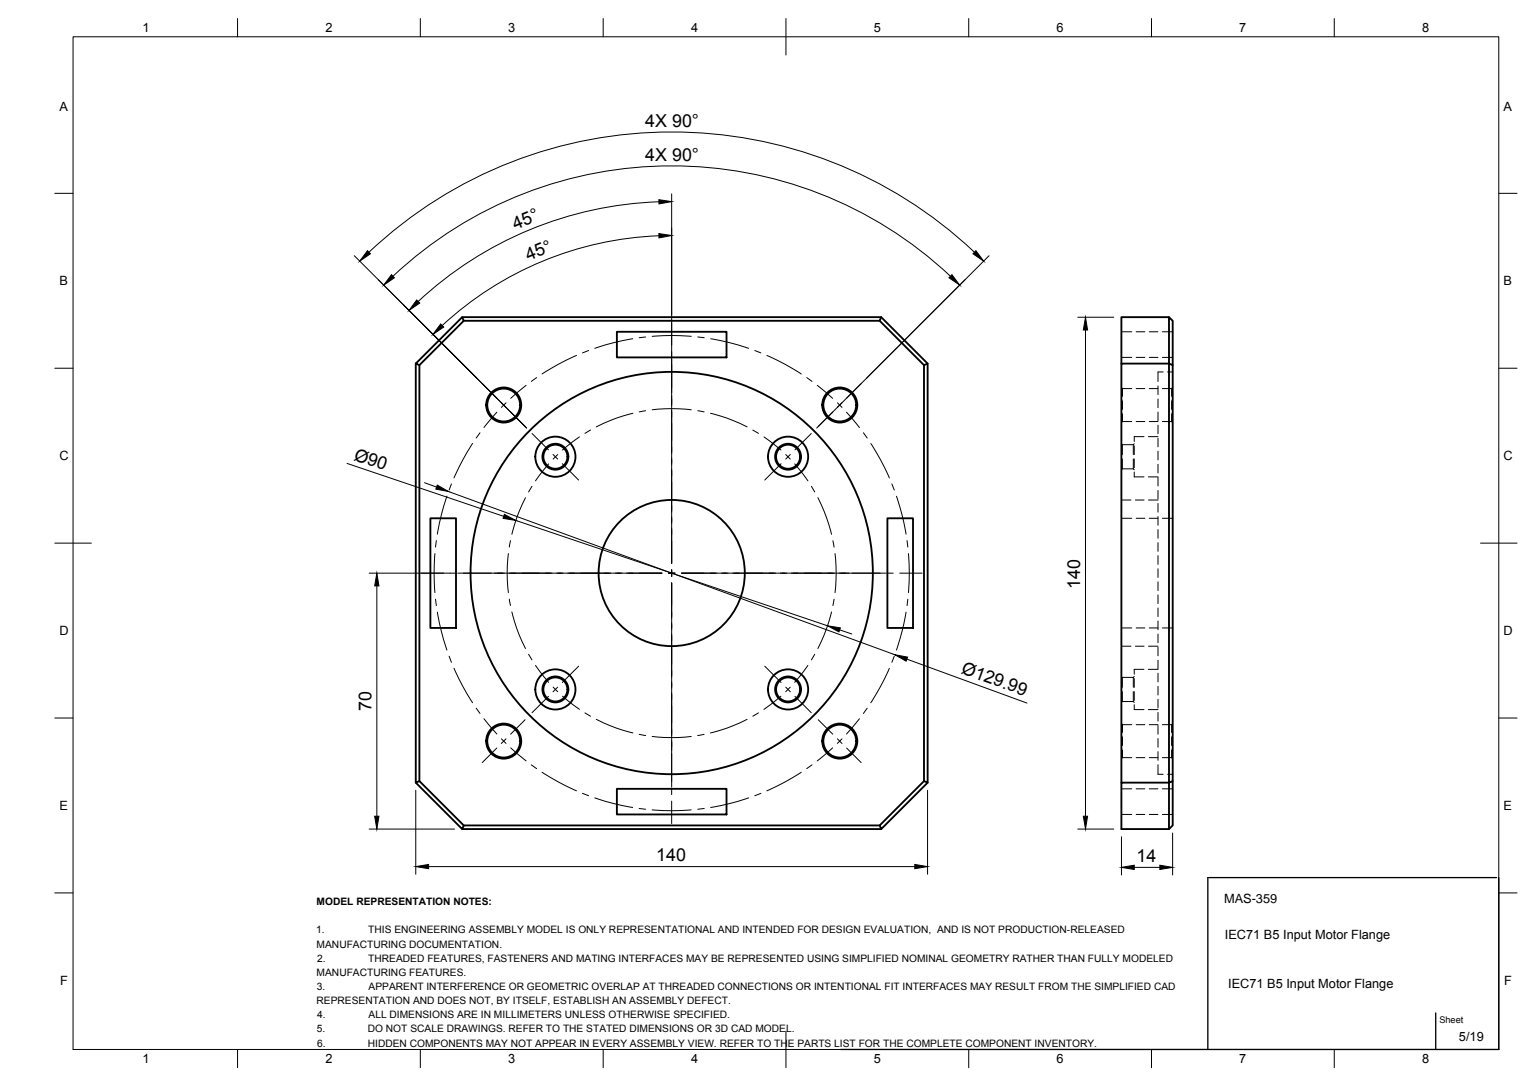
ISO-10303-21;
HEADER;
/* Generated by software containing ST-Developer
 * from STEP Tools, Inc. (www.steptools.com) 
 */

FILE_DESCRIPTION(
/* description */ (''),
/* implementation_level */ '2;1');

FILE_NAME(
/* name */ 'IEC71 B5 Input Motor Flange.step',
/* time_stamp */ '2026-10-15T14:25:16-07:00',
/* author */ (''),
/* organization */ (''),
/* preprocessor_version */ 'ST-DEVELOPER v20.2',
/* originating_system */ 'Autodesk Translation Framework v15.15.0.0',
/* authorisation */ '');

FILE_SCHEMA (('AUTOMOTIVE_DESIGN { 1 0 10303 214 3 1 1 }'));
ENDSEC;

DATA;
#10=MECHANICAL_DESIGN_GEOMETRIC_PRESENTATION_REPRESENTATION('',(#325),#86429);
#289=SHAPE_REPRESENTATION_RELATIONSHIP('SRR','None',#86504,#307);
#307=ADVANCED_BREP_SHAPE_REPRESENTATION('',(#343),#86413);
#325=STYLED_ITEM('',(#86603),#343);
#343=MANIFOLD_SOLID_BREP('Body1',#15615);
#1211=CONICAL_SURFACE('',#16324,0.3425,0.321750554396649);
#1212=CONICAL_SURFACE('',#16329,0.3425,0.785398163397466);
#1213=CONICAL_SURFACE('',#16335,0.3425,0.321750554396644);
#1214=CONICAL_SURFACE('',#16340,0.3425,0.785398163397457);
#1215=CONICAL_SURFACE('',#16346,0.3425,0.321750554396649);
#1216=CONICAL_SURFACE('',#16351,0.3425,0.785398163397466);
#1217=CONICAL_SURFACE('',#16357,0.3425,0.321750554396644);
#1218=CONICAL_SURFACE('',#16362,0.3425,0.785398163397457);
#1219=CONICAL_SURFACE('',#16368,0.49,0.785398163397448);
#1220=CONICAL_SURFACE('',#16373,0.49,0.785398163397443);
#1221=CONICAL_SURFACE('',#16374,0.49,0.785398163397448);
#1222=CONICAL_SURFACE('',#16379,0.49,0.785398163397443);
#1223=CONICAL_SURFACE('',#16380,0.49,0.785398163397448);
#1224=CONICAL_SURFACE('',#16385,0.49,0.785398163397443);
#1225=CONICAL_SURFACE('',#16386,0.49,0.785398163397448);
#1226=CONICAL_SURFACE('',#16391,0.49,0.785398163397443);
#1418=CYLINDRICAL_SURFACE('',#16327,0.33);
#1419=CYLINDRICAL_SURFACE('',#16333,0.55);
#1420=CYLINDRICAL_SURFACE('',#16338,0.33);
#1421=CYLINDRICAL_SURFACE('',#16344,0.55);
#1422=CYLINDRICAL_SURFACE('',#16349,0.33);
#1423=CYLINDRICAL_SURFACE('',#16355,0.55);
#1424=CYLINDRICAL_SURFACE('',#16360,0.33);
#1425=CYLINDRICAL_SURFACE('',#16366,0.55);
#1426=CYLINDRICAL_SURFACE('',#16371,0.45);
#1427=CYLINDRICAL_SURFACE('',#16377,0.45);
#1428=CYLINDRICAL_SURFACE('',#16383,0.45);
#1429=CYLINDRICAL_SURFACE('',#16389,0.45);
#1430=CYLINDRICAL_SURFACE('',#16408,2.);
#1431=CYLINDRICAL_SURFACE('',#16411,5.501);
#1668=FACE_BOUND('',#3613,.T.);
#1669=FACE_BOUND('',#3614,.T.);
#1670=FACE_BOUND('',#3615,.T.);
#1671=FACE_BOUND('',#3616,.T.);
#1672=FACE_BOUND('',#3617,.T.);
#1673=FACE_BOUND('',#3618,.T.);
#1674=FACE_BOUND('',#3619,.T.);
#1675=FACE_BOUND('',#3620,.T.);
#1676=FACE_BOUND('',#3621,.T.);
#1677=FACE_BOUND('',#3626,.T.);
#1678=FACE_BOUND('',#3632,.T.);
#1679=FACE_BOUND('',#3638,.T.);
#1680=FACE_BOUND('',#3644,.T.);
#1681=FACE_BOUND('',#3677,.T.);
#1682=FACE_BOUND('',#3678,.T.);
#1683=FACE_BOUND('',#3679,.T.);
#1684=FACE_BOUND('',#3680,.T.);
#1685=FACE_BOUND('',#3681,.T.);
#1686=FACE_BOUND('',#3687,.T.);
#1687=FACE_BOUND('',#3688,.T.);
#1688=FACE_BOUND('',#3689,.T.);
#1689=FACE_BOUND('',#3690,.T.);
#1690=FACE_BOUND('',#3691,.T.);
#1691=FACE_BOUND('',#3692,.T.);
#1692=FACE_BOUND('',#3693,.T.);
#1693=FACE_BOUND('',#3694,.T.);
#1694=FACE_BOUND('',#3695,.T.);
#1695=FACE_BOUND('',#3696,.T.);
#1696=FACE_BOUND('',#3697,.T.);
#1697=FACE_BOUND('',#3698,.T.);
#1698=FACE_BOUND('',#3699,.T.);
#1945=CIRCLE('',#16319,0.480000000000001);
#1946=CIRCLE('',#16320,5.501);
#1947=CIRCLE('',#16321,0.480000000000001);
#1948=CIRCLE('',#16322,0.480000000000001);
#1949=CIRCLE('',#16323,0.480000000000001);
#1950=CIRCLE('',#16325,0.33);
#1951=CIRCLE('',#16326,0.338333333333333);
#1952=CIRCLE('',#16328,0.33);
#1953=CIRCLE('',#16330,0.355);
#1954=CIRCLE('',#16332,0.55);
#1955=CIRCLE('',#16334,0.55);
#1956=CIRCLE('',#16336,0.33);
#1957=CIRCLE('',#16337,0.338333333333333);
#1958=CIRCLE('',#16339,0.33);
#1959=CIRCLE('',#16341,0.355);
#1960=CIRCLE('',#16343,0.55);
#1961=CIRCLE('',#16345,0.55);
#1962=CIRCLE('',#16347,0.33);
#1963=CIRCLE('',#16348,0.338333333333333);
#1964=CIRCLE('',#16350,0.33);
#1965=CIRCLE('',#16352,0.355);
#1966=CIRCLE('',#16354,0.55);
#1967=CIRCLE('',#16356,0.55);
#1968=CIRCLE('',#16358,0.33);
#1969=CIRCLE('',#16359,0.338333333333333);
#1970=CIRCLE('',#16361,0.33);
#1971=CIRCLE('',#16363,0.355);
#1972=CIRCLE('',#16365,0.55);
#1973=CIRCLE('',#16367,0.55);
#1974=CIRCLE('',#16369,0.45);
#1975=CIRCLE('',#16370,0.48);
#1976=CIRCLE('',#16372,0.45);
#1977=CIRCLE('',#16375,0.45);
#1978=CIRCLE('',#16376,0.48);
#1979=CIRCLE('',#16378,0.45);
#1980=CIRCLE('',#16381,0.45);
#1981=CIRCLE('',#16382,0.48);
#1982=CIRCLE('',#16384,0.45);
#1983=CIRCLE('',#16387,0.45);
#1984=CIRCLE('',#16388,0.48);
#1985=CIRCLE('',#16390,0.45);
#1986=CIRCLE('',#16409,2.);
#1987=CIRCLE('',#16410,2.);
#1988=CIRCLE('',#16412,5.501);
#2662=FACE_OUTER_BOUND('',#3600,.T.);
#2663=FACE_OUTER_BOUND('',#3601,.T.);
#2664=FACE_OUTER_BOUND('',#3602,.T.);
#2665=FACE_OUTER_BOUND('',#3603,.T.);
#2666=FACE_OUTER_BOUND('',#3604,.T.);
#2667=FACE_OUTER_BOUND('',#3605,.T.);
#2668=FACE_OUTER_BOUND('',#3606,.T.);
#2669=FACE_OUTER_BOUND('',#3607,.T.);
#2670=FACE_OUTER_BOUND('',#3608,.T.);
#2671=FACE_OUTER_BOUND('',#3609,.T.);
#2672=FACE_OUTER_BOUND('',#3610,.T.);
#2673=FACE_OUTER_BOUND('',#3611,.T.);
#2674=FACE_OUTER_BOUND('',#3612,.T.);
#2675=FACE_OUTER_BOUND('',#3622,.T.);
#2676=FACE_OUTER_BOUND('',#3623,.T.);
#2677=FACE_OUTER_BOUND('',#3624,.T.);
#2678=FACE_OUTER_BOUND('',#3625,.T.);
#2679=FACE_OUTER_BOUND('',#3627,.T.);
#2680=FACE_OUTER_BOUND('',#3628,.T.);
#2681=FACE_OUTER_BOUND('',#3629,.T.);
#2682=FACE_OUTER_BOUND('',#3630,.T.);
#2683=FACE_OUTER_BOUND('',#3631,.T.);
#2684=FACE_OUTER_BOUND('',#3633,.T.);
#2685=FACE_OUTER_BOUND('',#3634,.T.);
#2686=FACE_OUTER_BOUND('',#3635,.T.);
#2687=FACE_OUTER_BOUND('',#3636,.T.);
#2688=FACE_OUTER_BOUND('',#3637,.T.);
#2689=FACE_OUTER_BOUND('',#3639,.T.);
#2690=FACE_OUTER_BOUND('',#3640,.T.);
#2691=FACE_OUTER_BOUND('',#3641,.T.);
#2692=FACE_OUTER_BOUND('',#3642,.T.);
#2693=FACE_OUTER_BOUND('',#3643,.T.);
#2694=FACE_OUTER_BOUND('',#3645,.T.);
#2695=FACE_OUTER_BOUND('',#3646,.T.);
#2696=FACE_OUTER_BOUND('',#3647,.T.);
#2697=FACE_OUTER_BOUND('',#3648,.T.);
#2698=FACE_OUTER_BOUND('',#3649,.T.);
#2699=FACE_OUTER_BOUND('',#3650,.T.);
#2700=FACE_OUTER_BOUND('',#3651,.T.);
#2701=FACE_OUTER_BOUND('',#3652,.T.);
#2702=FACE_OUTER_BOUND('',#3653,.T.);
#2703=FACE_OUTER_BOUND('',#3654,.T.);
#2704=FACE_OUTER_BOUND('',#3655,.T.);
#2705=FACE_OUTER_BOUND('',#3656,.T.);
#2706=FACE_OUTER_BOUND('',#3657,.T.);
#2707=FACE_OUTER_BOUND('',#3658,.T.);
#2708=FACE_OUTER_BOUND('',#3659,.T.);
#2709=FACE_OUTER_BOUND('',#3660,.T.);
#2710=FACE_OUTER_BOUND('',#3661,.T.);
#2711=FACE_OUTER_BOUND('',#3662,.T.);
#2712=FACE_OUTER_BOUND('',#3663,.T.);
#2713=FACE_OUTER_BOUND('',#3664,.T.);
#2714=FACE_OUTER_BOUND('',#3665,.T.);
#2715=FACE_OUTER_BOUND('',#3666,.T.);
#2716=FACE_OUTER_BOUND('',#3667,.T.);
#2717=FACE_OUTER_BOUND('',#3668,.T.);
#2718=FACE_OUTER_BOUND('',#3669,.T.);
#2719=FACE_OUTER_BOUND('',#3670,.T.);
#2720=FACE_OUTER_BOUND('',#3671,.T.);
#2721=FACE_OUTER_BOUND('',#3672,.T.);
#2722=FACE_OUTER_BOUND('',#3673,.T.);
#2723=FACE_OUTER_BOUND('',#3674,.T.);
#2724=FACE_OUTER_BOUND('',#3675,.T.);
#2725=FACE_OUTER_BOUND('',#3676,.T.);
#2726=FACE_OUTER_BOUND('',#3682,.T.);
#2727=FACE_OUTER_BOUND('',#3683,.T.);
#2728=FACE_OUTER_BOUND('',#3684,.T.);
#2729=FACE_OUTER_BOUND('',#3685,.T.);
#2730=FACE_OUTER_BOUND('',#3686,.T.);
#3600=EDGE_LOOP('',(#11207,#11208,#11209,#11210));
#3601=EDGE_LOOP('',(#11211,#11212,#11213,#11214));
#3602=EDGE_LOOP('',(#11215,#11216,#11217,#11218));
#3603=EDGE_LOOP('',(#11219,#11220,#11221,#11222));
#3604=EDGE_LOOP('',(#11223,#11224,#11225,#11226));
#3605=EDGE_LOOP('',(#11227,#11228,#11229,#11230));
#3606=EDGE_LOOP('',(#11231,#11232,#11233,#11234));
#3607=EDGE_LOOP('',(#11235,#11236,#11237,#11238));
#3608=EDGE_LOOP('',(#11239,#11240,#11241,#11242));
#3609=EDGE_LOOP('',(#11243,#11244,#11245,#11246));
#3610=EDGE_LOOP('',(#11247,#11248,#11249,#11250));
#3611=EDGE_LOOP('',(#11251,#11252,#11253,#11254));
#3612=EDGE_LOOP('',(#11255,#11256,#11257,#11258,#11259,#11260,#11261,#11262));
#3613=EDGE_LOOP('',(#11263));
#3614=EDGE_LOOP('',(#11264,#11265,#11266,#11267));
#3615=EDGE_LOOP('',(#11268,#11269,#11270,#11271));
#3616=EDGE_LOOP('',(#11272,#11273,#11274,#11275));
#3617=EDGE_LOOP('',(#11276,#11277,#11278,#11279));
#3618=EDGE_LOOP('',(#11280));
#3619=EDGE_LOOP('',(#11281));
#3620=EDGE_LOOP('',(#11282));
#3621=EDGE_LOOP('',(#11283));
#3622=EDGE_LOOP('',(#11284,#11285,#11286,#11287));
#3623=EDGE_LOOP('',(#11288,#11289,#11290,#11291));
#3624=EDGE_LOOP('',(#11292,#11293,#11294,#11295));
#3625=EDGE_LOOP('',(#11296));
#3626=EDGE_LOOP('',(#11297));
#3627=EDGE_LOOP('',(#11298,#11299,#11300,#11301));
#3628=EDGE_LOOP('',(#11302,#11303,#11304,#11305));
#3629=EDGE_LOOP('',(#11306,#11307,#11308,#11309));
#3630=EDGE_LOOP('',(#11310,#11311,#11312,#11313));
#3631=EDGE_LOOP('',(#11314));
#3632=EDGE_LOOP('',(#11315));
#3633=EDGE_LOOP('',(#11316,#11317,#11318,#11319));
#3634=EDGE_LOOP('',(#11320,#11321,#11322,#11323));
#3635=EDGE_LOOP('',(#11324,#11325,#11326,#11327));
#3636=EDGE_LOOP('',(#11328,#11329,#11330,#11331));
#3637=EDGE_LOOP('',(#11332));
#3638=EDGE_LOOP('',(#11333));
#3639=EDGE_LOOP('',(#11334,#11335,#11336,#11337));
#3640=EDGE_LOOP('',(#11338,#11339,#11340,#11341));
#3641=EDGE_LOOP('',(#11342,#11343,#11344,#11345));
#3642=EDGE_LOOP('',(#11346,#11347,#11348,#11349));
#3643=EDGE_LOOP('',(#11350));
#3644=EDGE_LOOP('',(#11351));
#3645=EDGE_LOOP('',(#11352,#11353,#11354,#11355));
#3646=EDGE_LOOP('',(#11356,#11357,#11358,#11359));
#3647=EDGE_LOOP('',(#11360,#11361,#11362,#11363));
#3648=EDGE_LOOP('',(#11364,#11365,#11366,#11367));
#3649=EDGE_LOOP('',(#11368,#11369,#11370,#11371));
#3650=EDGE_LOOP('',(#11372,#11373,#11374,#11375));
#3651=EDGE_LOOP('',(#11376,#11377,#11378,#11379));
#3652=EDGE_LOOP('',(#11380,#11381,#11382,#11383));
#3653=EDGE_LOOP('',(#11384,#11385,#11386,#11387));
#3654=EDGE_LOOP('',(#11388,#11389,#11390,#11391));
#3655=EDGE_LOOP('',(#11392,#11393,#11394,#11395));
#3656=EDGE_LOOP('',(#11396,#11397,#11398,#11399));
#3657=EDGE_LOOP('',(#11400,#11401,#11402,#11403));
#3658=EDGE_LOOP('',(#11404,#11405,#11406,#11407));
#3659=EDGE_LOOP('',(#11408,#11409,#11410,#11411));
#3660=EDGE_LOOP('',(#11412,#11413,#11414,#11415));
#3661=EDGE_LOOP('',(#11416,#11417,#11418,#11419));
#3662=EDGE_LOOP('',(#11420,#11421,#11422,#11423));
#3663=EDGE_LOOP('',(#11424,#11425,#11426,#11427));
#3664=EDGE_LOOP('',(#11428,#11429,#11430,#11431));
#3665=EDGE_LOOP('',(#11432,#11433,#11434,#11435));
#3666=EDGE_LOOP('',(#11436,#11437,#11438,#11439));
#3667=EDGE_LOOP('',(#11440,#11441,#11442,#11443));
#3668=EDGE_LOOP('',(#11444,#11445,#11446,#11447));
#3669=EDGE_LOOP('',(#11448,#11449,#11450,#11451));
#3670=EDGE_LOOP('',(#11452,#11453,#11454,#11455));
#3671=EDGE_LOOP('',(#11456,#11457,#11458,#11459));
#3672=EDGE_LOOP('',(#11460,#11461,#11462,#11463));
#3673=EDGE_LOOP('',(#11464,#11465,#11466,#11467));
#3674=EDGE_LOOP('',(#11468,#11469,#11470,#11471));
#3675=EDGE_LOOP('',(#11472,#11473,#11474,#11475));
#3676=EDGE_LOOP('',(#11476));
#3677=EDGE_LOOP('',(#11477));
#3678=EDGE_LOOP('',(#11478));
#3679=EDGE_LOOP('',(#11479));
#3680=EDGE_LOOP('',(#11480));
#3681=EDGE_LOOP('',(#11481));
#3682=EDGE_LOOP('',(#11482,#11483,#11484,#11485));
#3683=EDGE_LOOP('',(#11486,#11487,#11488,#11489));
#3684=EDGE_LOOP('',(#11490,#11491,#11492,#11493));
#3685=EDGE_LOOP('',(#11494,#11495,#11496,#11497));
#3686=EDGE_LOOP('',(#11498,#11499,#11500,#11501,#11502,#11503,#11504,#11505));
#3687=EDGE_LOOP('',(#11506));
#3688=EDGE_LOOP('',(#11507));
#3689=EDGE_LOOP('',(#11508));
#3690=EDGE_LOOP('',(#11509));
#3691=EDGE_LOOP('',(#11510));
#3692=EDGE_LOOP('',(#11511));
#3693=EDGE_LOOP('',(#11512,#11513,#11514,#11515));
#3694=EDGE_LOOP('',(#11516,#11517,#11518,#11519));
#3695=EDGE_LOOP('',(#11520,#11521,#11522,#11523));
#3696=EDGE_LOOP('',(#11524,#11525,#11526,#11527));
#3697=EDGE_LOOP('',(#11528));
#3698=EDGE_LOOP('',(#11529));
#3699=EDGE_LOOP('',(#11530));
#4732=LINE('',#22793,#5592);
#4733=LINE('',#22795,#5593);
#4734=LINE('',#22797,#5594);
#4735=LINE('',#22798,#5595);
#4736=LINE('',#22801,#5596);
#4737=LINE('',#22803,#5597);
#4738=LINE('',#22804,#5598);
#4739=LINE('',#22807,#5599);
#4740=LINE('',#22809,#5600);
#4741=LINE('',#22810,#5601);
#4742=LINE('',#22813,#5602);
#4743=LINE('',#22815,#5603);
#4744=LINE('',#22816,#5604);
#4745=LINE('',#22819,#5605);
#4746=LINE('',#22821,#5606);
#4747=LINE('',#22822,#5607);
#4748=LINE('',#22825,#5608);
#4749=LINE('',#22827,#5609);
#4750=LINE('',#22828,#5610);
#4751=LINE('',#22831,#5611);
#4752=LINE('',#22833,#5612);
#4753=LINE('',#22834,#5613);
#4754=LINE('',#22836,#5614);
#4755=LINE('',#22837,#5615);
#4756=LINE('',#22840,#5616);
#4757=LINE('',#22842,#5617);
#4758=LINE('',#22843,#5618);
#4759=LINE('',#22846,#5619);
#4760=LINE('',#22847,#5620);
#4761=LINE('',#22850,#5621);
#4762=LINE('',#22851,#5622);
#4763=LINE('',#22854,#5623);
#4764=LINE('',#22855,#5624);
#4765=LINE('',#22861,#5625);
#4766=LINE('',#22863,#5626);
#4767=LINE('',#22865,#5627);
#4768=LINE('',#22866,#5628);
#4769=LINE('',#22869,#5629);
#4770=LINE('',#22871,#5630);
#4771=LINE('',#22873,#5631);
#4772=LINE('',#22874,#5632);
#4773=LINE('',#22877,#5633);
#4774=LINE('',#22879,#5634);
#4775=LINE('',#22881,#5635);
#4776=LINE('',#22882,#5636);
#4777=LINE('',#22885,#5637);
#4778=LINE('',#22887,#5638);
#4779=LINE('',#22889,#5639);
#4780=LINE('',#22890,#5640);
#4781=LINE('',#22903,#5641);
#4782=LINE('',#22907,#5642);
#4783=LINE('',#22911,#5643);
#4784=LINE('',#22918,#5644);
#4785=LINE('',#22924,#5645);
#4786=LINE('',#22928,#5646);
#4787=LINE('',#22932,#5647);
#4788=LINE('',#22939,#5648);
#4789=LINE('',#22945,#5649);
#4790=LINE('',#22949,#5650);
#4791=LINE('',#22953,#5651);
#4792=LINE('',#22960,#5652);
#4793=LINE('',#22966,#5653);
#4794=LINE('',#22970,#5654);
#4795=LINE('',#22974,#5655);
#4796=LINE('',#22981,#5656);
#4797=LINE('',#22987,#5657);
#4798=LINE('',#22991,#5658);
#4799=LINE('',#22994,#5659);
#4800=LINE('',#22999,#5660);
#4801=LINE('',#23003,#5661);
#4802=LINE('',#23006,#5662);
#4803=LINE('',#23011,#5663);
#4804=LINE('',#23015,#5664);
#4805=LINE('',#23018,#5665);
#4806=LINE('',#23023,#5666);
#4807=LINE('',#23027,#5667);
#4808=LINE('',#23030,#5668);
#4809=LINE('',#23034,#5669);
#4810=LINE('',#23035,#5670);
#4811=LINE('',#23036,#5671);
#4812=LINE('',#23039,#5672);
#4813=LINE('',#23040,#5673);
#4814=LINE('',#23043,#5674);
#4815=LINE('',#23044,#5675);
#4816=LINE('',#23046,#5676);
#4817=LINE('',#23050,#5677);
#4818=LINE('',#23051,#5678);
#4819=LINE('',#23052,#5679);
#4820=LINE('',#23055,#5680);
#4821=LINE('',#23056,#5681);
#4822=LINE('',#23059,#5682);
#4823=LINE('',#23060,#5683);
#4824=LINE('',#23062,#5684);
#4825=LINE('',#23066,#5685);
#4826=LINE('',#23067,#5686);
#4827=LINE('',#23068,#5687);
#4828=LINE('',#23071,#5688);
#4829=LINE('',#23072,#5689);
#4830=LINE('',#23075,#5690);
#4831=LINE('',#23076,#5691);
#4832=LINE('',#23078,#5692);
#4833=LINE('',#23082,#5693);
#4834=LINE('',#23083,#5694);
#4835=LINE('',#23084,#5695);
#4836=LINE('',#23087,#5696);
#4837=LINE('',#23088,#5697);
#4838=LINE('',#23091,#5698);
#4839=LINE('',#23092,#5699);
#4840=LINE('',#23094,#5700);
#4841=LINE('',#23099,#5701);
#4842=LINE('',#23103,#5702);
#4843=LINE('',#23108,#5703);
#4844=LINE('',#23109,#5704);
#4845=LINE('',#23112,#5705);
#4846=LINE('',#23113,#5706);
#4847=LINE('',#23116,#5707);
#4848=LINE('',#23117,#5708);
#4849=LINE('',#23119,#5709);
#5592=VECTOR('',#18691,1.);
#5593=VECTOR('',#18692,1.);
#5594=VECTOR('',#18693,1.);
#5595=VECTOR('',#18694,0.999999999999999);
#5596=VECTOR('',#18697,1.);
#5597=VECTOR('',#18698,1.);
#5598=VECTOR('',#18699,1.);
#5599=VECTOR('',#18702,1.);
#5600=VECTOR('',#18703,1.);
#5601=VECTOR('',#18704,1.);
#5602=VECTOR('',#18707,1.);
#5603=VECTOR('',#18708,0.999999999999999);
#5604=VECTOR('',#18709,1.);
#5605=VECTOR('',#18712,1.);
#5606=VECTOR('',#18713,0.999999999999999);
#5607=VECTOR('',#18714,1.);
#5608=VECTOR('',#18717,1.);
#5609=VECTOR('',#18718,1.);
#5610=VECTOR('',#18719,1.);
#5611=VECTOR('',#18722,1.);
#5612=VECTOR('',#18723,1.);
#5613=VECTOR('',#18724,1.);
#5614=VECTOR('',#18727,1.);
#5615=VECTOR('',#18728,1.);
#5616=VECTOR('',#18731,1.);
#5617=VECTOR('',#18732,1.);
#5618=VECTOR('',#18733,1.);
#5619=VECTOR('',#18736,1.);
#5620=VECTOR('',#18737,1.);
#5621=VECTOR('',#18740,1.);
#5622=VECTOR('',#18741,1.);
#5623=VECTOR('',#18744,1.);
#5624=VECTOR('',#18745,1.);
#5625=VECTOR('',#18750,1.);
#5626=VECTOR('',#18751,1.);
#5627=VECTOR('',#18752,1.);
#5628=VECTOR('',#18753,1.);
#5629=VECTOR('',#18754,1.);
#5630=VECTOR('',#18755,1.);
#5631=VECTOR('',#18756,1.);
#5632=VECTOR('',#18757,1.);
#5633=VECTOR('',#18758,1.);
#5634=VECTOR('',#18759,1.);
#5635=VECTOR('',#18760,1.);
#5636=VECTOR('',#18761,1.);
#5637=VECTOR('',#18762,1.);
#5638=VECTOR('',#18763,1.);
#5639=VECTOR('',#18764,1.);
#5640=VECTOR('',#18765,1.);
#5641=VECTOR('',#18778,0.3425);
#5642=VECTOR('',#18783,0.33);
#5643=VECTOR('',#18788,0.3425);
#5644=VECTOR('',#18797,0.55);
#5645=VECTOR('',#18804,0.3425);
#5646=VECTOR('',#18809,0.33);
#5647=VECTOR('',#18814,0.3425);
#5648=VECTOR('',#18823,0.55);
#5649=VECTOR('',#18830,0.3425);
#5650=VECTOR('',#18835,0.33);
#5651=VECTOR('',#18840,0.3425);
#5652=VECTOR('',#18849,0.55);
#5653=VECTOR('',#18856,0.3425);
#5654=VECTOR('',#18861,0.33);
#5655=VECTOR('',#18866,0.3425);
#5656=VECTOR('',#18875,0.55);
#5657=VECTOR('',#18882,0.49);
#5658=VECTOR('',#18887,0.45);
#5659=VECTOR('',#18892,0.49);
#5660=VECTOR('',#18897,0.49);
#5661=VECTOR('',#18902,0.45);
#5662=VECTOR('',#18907,0.49);
#5663=VECTOR('',#18912,0.49);
#5664=VECTOR('',#18917,0.45);
#5665=VECTOR('',#18922,0.49);
#5666=VECTOR('',#18927,0.49);
#5667=VECTOR('',#18932,0.45);
#5668=VECTOR('',#18937,0.49);
#5669=VECTOR('',#18940,1.);
#5670=VECTOR('',#18941,1.);
#5671=VECTOR('',#18942,1.);
#5672=VECTOR('',#18945,1.);
#5673=VECTOR('',#18946,1.);
#5674=VECTOR('',#18949,1.);
#5675=VECTOR('',#18950,1.);
#5676=VECTOR('',#18953,1.);
#5677=VECTOR('',#18956,1.);
#5678=VECTOR('',#18957,1.);
#5679=VECTOR('',#18958,1.);
#5680=VECTOR('',#18961,1.);
#5681=VECTOR('',#18962,1.);
#5682=VECTOR('',#18965,1.);
#5683=VECTOR('',#18966,1.);
#5684=VECTOR('',#18969,1.);
#5685=VECTOR('',#18972,1.);
#5686=VECTOR('',#18973,1.);
#5687=VECTOR('',#18974,1.);
#5688=VECTOR('',#18977,1.);
#5689=VECTOR('',#18978,1.);
#5690=VECTOR('',#18981,1.);
#5691=VECTOR('',#18982,1.);
#5692=VECTOR('',#18985,1.);
#5693=VECTOR('',#18988,1.);
#5694=VECTOR('',#18989,1.);
#5695=VECTOR('',#18990,1.);
#5696=VECTOR('',#18993,1.);
#5697=VECTOR('',#18994,1.);
#5698=VECTOR('',#18997,1.);
#5699=VECTOR('',#18998,1.);
#5700=VECTOR('',#19001,1.);
#5701=VECTOR('',#19006,2.);
#5702=VECTOR('',#19011,5.501);
#5703=VECTOR('',#19018,1.);
#5704=VECTOR('',#19019,1.);
#5705=VECTOR('',#19022,1.);
#5706=VECTOR('',#19023,1.);
#5707=VECTOR('',#19026,1.);
#5708=VECTOR('',#19027,1.);
#5709=VECTOR('',#19030,1.);
#6442=VERTEX_POINT('',#22791);
#6443=VERTEX_POINT('',#22792);
#6444=VERTEX_POINT('',#22794);
#6445=VERTEX_POINT('',#22796);
#6446=VERTEX_POINT('',#22800);
#6447=VERTEX_POINT('',#22802);
#6448=VERTEX_POINT('',#22806);
#6449=VERTEX_POINT('',#22808);
#6450=VERTEX_POINT('',#22812);
#6451=VERTEX_POINT('',#22814);
#6452=VERTEX_POINT('',#22818);
#6453=VERTEX_POINT('',#22820);
#6454=VERTEX_POINT('',#22824);
#6455=VERTEX_POINT('',#22826);
#6456=VERTEX_POINT('',#22830);
#6457=VERTEX_POINT('',#22832);
#6458=VERTEX_POINT('',#22839);
#6459=VERTEX_POINT('',#22841);
#6460=VERTEX_POINT('',#22845);
#6461=VERTEX_POINT('',#22849);
#6462=VERTEX_POINT('',#22853);
#6463=VERTEX_POINT('',#22857);
#6464=VERTEX_POINT('',#22859);
#6465=VERTEX_POINT('',#22860);
#6466=VERTEX_POINT('',#22862);
#6467=VERTEX_POINT('',#22864);
#6468=VERTEX_POINT('',#22867);
#6469=VERTEX_POINT('',#22868);
#6470=VERTEX_POINT('',#22870);
#6471=VERTEX_POINT('',#22872);
#6472=VERTEX_POINT('',#22875);
#6473=VERTEX_POINT('',#22876);
#6474=VERTEX_POINT('',#22878);
#6475=VERTEX_POINT('',#22880);
#6476=VERTEX_POINT('',#22883);
#6477=VERTEX_POINT('',#22884);
#6478=VERTEX_POINT('',#22886);
#6479=VERTEX_POINT('',#22888);
#6480=VERTEX_POINT('',#22891);
#6481=VERTEX_POINT('',#22893);
#6482=VERTEX_POINT('',#22895);
#6483=VERTEX_POINT('',#22897);
#6484=VERTEX_POINT('',#22900);
#6485=VERTEX_POINT('',#22902);
#6486=VERTEX_POINT('',#22906);
#6487=VERTEX_POINT('',#22910);
#6488=VERTEX_POINT('',#22914);
#6489=VERTEX_POINT('',#22917);
#6490=VERTEX_POINT('',#22921);
#6491=VERTEX_POINT('',#22923);
#6492=VERTEX_POINT('',#22927);
#6493=VERTEX_POINT('',#22931);
#6494=VERTEX_POINT('',#22935);
#6495=VERTEX_POINT('',#22938);
#6496=VERTEX_POINT('',#22942);
#6497=VERTEX_POINT('',#22944);
#6498=VERTEX_POINT('',#22948);
#6499=VERTEX_POINT('',#22952);
#6500=VERTEX_POINT('',#22956);
#6501=VERTEX_POINT('',#22959);
#6502=VERTEX_POINT('',#22963);
#6503=VERTEX_POINT('',#22965);
#6504=VERTEX_POINT('',#22969);
#6505=VERTEX_POINT('',#22973);
#6506=VERTEX_POINT('',#22977);
#6507=VERTEX_POINT('',#22980);
#6508=VERTEX_POINT('',#22984);
#6509=VERTEX_POINT('',#22986);
#6510=VERTEX_POINT('',#22990);
#6511=VERTEX_POINT('',#22996);
#6512=VERTEX_POINT('',#22998);
#6513=VERTEX_POINT('',#23002);
#6514=VERTEX_POINT('',#23008);
#6515=VERTEX_POINT('',#23010);
#6516=VERTEX_POINT('',#23014);
#6517=VERTEX_POINT('',#23020);
#6518=VERTEX_POINT('',#23022);
#6519=VERTEX_POINT('',#23026);
#6520=VERTEX_POINT('',#23032);
#6521=VERTEX_POINT('',#23033);
#6522=VERTEX_POINT('',#23038);
#6523=VERTEX_POINT('',#23042);
#6524=VERTEX_POINT('',#23048);
#6525=VERTEX_POINT('',#23049);
#6526=VERTEX_POINT('',#23054);
#6527=VERTEX_POINT('',#23058);
#6528=VERTEX_POINT('',#23064);
#6529=VERTEX_POINT('',#23065);
#6530=VERTEX_POINT('',#23070);
#6531=VERTEX_POINT('',#23074);
#6532=VERTEX_POINT('',#23080);
#6533=VERTEX_POINT('',#23081);
#6534=VERTEX_POINT('',#23086);
#6535=VERTEX_POINT('',#23090);
#6536=VERTEX_POINT('',#23096);
#6537=VERTEX_POINT('',#23098);
#6538=VERTEX_POINT('',#23102);
#6539=VERTEX_POINT('',#23107);
#6540=VERTEX_POINT('',#23111);
#6541=VERTEX_POINT('',#23115);
#8225=EDGE_CURVE('',#6442,#6443,#4732,.T.);
#8226=EDGE_CURVE('',#6443,#6444,#4733,.T.);
#8227=EDGE_CURVE('',#6444,#6445,#4734,.T.);
#8228=EDGE_CURVE('',#6442,#6445,#4735,.T.);
#8229=EDGE_CURVE('',#6443,#6446,#4736,.T.);
#8230=EDGE_CURVE('',#6446,#6447,#4737,.T.);
#8231=EDGE_CURVE('',#6447,#6444,#4738,.T.);
#8232=EDGE_CURVE('',#6446,#6448,#4739,.T.);
#8233=EDGE_CURVE('',#6448,#6449,#4740,.T.);
#8234=EDGE_CURVE('',#6449,#6447,#4741,.T.);
#8235=EDGE_CURVE('',#6448,#6450,#4742,.T.);
#8236=EDGE_CURVE('',#6450,#6451,#4743,.T.);
#8237=EDGE_CURVE('',#6451,#6449,#4744,.T.);
#8238=EDGE_CURVE('',#6450,#6452,#4745,.T.);
#8239=EDGE_CURVE('',#6452,#6453,#4746,.T.);
#8240=EDGE_CURVE('',#6453,#6451,#4747,.T.);
#8241=EDGE_CURVE('',#6454,#6453,#4748,.T.);
#8242=EDGE_CURVE('',#6452,#6455,#4749,.T.);
#8243=EDGE_CURVE('',#6455,#6454,#4750,.T.);
#8244=EDGE_CURVE('',#6456,#6454,#4751,.T.);
#8245=EDGE_CURVE('',#6455,#6457,#4752,.T.);
#8246=EDGE_CURVE('',#6457,#6456,#4753,.T.);
#8247=EDGE_CURVE('',#6445,#6456,#4754,.T.);
#8248=EDGE_CURVE('',#6457,#6442,#4755,.T.);
#8249=EDGE_CURVE('',#6458,#6454,#4756,.T.);
#8250=EDGE_CURVE('',#6459,#6458,#4757,.T.);
#8251=EDGE_CURVE('',#6459,#6453,#4758,.T.);
#8252=EDGE_CURVE('',#6460,#6456,#4759,.T.);
#8253=EDGE_CURVE('',#6458,#6460,#4760,.T.);
#8254=EDGE_CURVE('',#6461,#6445,#4761,.T.);
#8255=EDGE_CURVE('',#6460,#6461,#4762,.T.);
#8256=EDGE_CURVE('',#6462,#6444,#4763,.T.);
#8257=EDGE_CURVE('',#6461,#6462,#4764,.T.);
#8258=EDGE_CURVE('',#6463,#6463,#1945,.T.);
#8259=EDGE_CURVE('',#6464,#6465,#4765,.T.);
#8260=EDGE_CURVE('',#6465,#6466,#4766,.T.);
#8261=EDGE_CURVE('',#6466,#6467,#4767,.T.);
#8262=EDGE_CURVE('',#6467,#6464,#4768,.T.);
#8263=EDGE_CURVE('',#6468,#6469,#4769,.T.);
#8264=EDGE_CURVE('',#6469,#6470,#4770,.T.);
#8265=EDGE_CURVE('',#6470,#6471,#4771,.T.);
#8266=EDGE_CURVE('',#6471,#6468,#4772,.T.);
#8267=EDGE_CURVE('',#6472,#6473,#4773,.T.);
#8268=EDGE_CURVE('',#6473,#6474,#4774,.T.);
#8269=EDGE_CURVE('',#6474,#6475,#4775,.T.);
#8270=EDGE_CURVE('',#6475,#6472,#4776,.T.);
#8271=EDGE_CURVE('',#6476,#6477,#4777,.T.);
#8272=EDGE_CURVE('',#6477,#6478,#4778,.T.);
#8273=EDGE_CURVE('',#6478,#6479,#4779,.T.);
#8274=EDGE_CURVE('',#6479,#6476,#4780,.T.);
#8275=EDGE_CURVE('',#6480,#6480,#1946,.T.);
#8276=EDGE_CURVE('',#6481,#6481,#1947,.T.);
#8277=EDGE_CURVE('',#6482,#6482,#1948,.T.);
#8278=EDGE_CURVE('',#6483,#6483,#1949,.T.);
#8279=EDGE_CURVE('',#6484,#6484,#1950,.T.);
#8280=EDGE_CURVE('',#6484,#6485,#4781,.T.);
#8281=EDGE_CURVE('',#6485,#6485,#1951,.T.);
#8282=EDGE_CURVE('',#6484,#6486,#4782,.T.);
#8283=EDGE_CURVE('',#6486,#6486,#1952,.T.);
#8284=EDGE_CURVE('',#6486,#6487,#4783,.T.);
#8285=EDGE_CURVE('',#6487,#6487,#1953,.T.);
#8286=EDGE_CURVE('',#6488,#6488,#1954,.T.);
#8287=EDGE_CURVE('',#6488,#6489,#4784,.T.);
#8288=EDGE_CURVE('',#6489,#6489,#1955,.T.);
#8289=EDGE_CURVE('',#6490,#6490,#1956,.T.);
#8290=EDGE_CURVE('',#6490,#6491,#4785,.T.);
#8291=EDGE_CURVE('',#6491,#6491,#1957,.T.);
#8292=EDGE_CURVE('',#6490,#6492,#4786,.T.);
#8293=EDGE_CURVE('',#6492,#6492,#1958,.T.);
#8294=EDGE_CURVE('',#6492,#6493,#4787,.T.);
#8295=EDGE_CURVE('',#6493,#6493,#1959,.T.);
#8296=EDGE_CURVE('',#6494,#6494,#1960,.T.);
#8297=EDGE_CURVE('',#6494,#6495,#4788,.T.);
#8298=EDGE_CURVE('',#6495,#6495,#1961,.T.);
#8299=EDGE_CURVE('',#6496,#6496,#1962,.T.);
#8300=EDGE_CURVE('',#6496,#6497,#4789,.T.);
#8301=EDGE_CURVE('',#6497,#6497,#1963,.T.);
#8302=EDGE_CURVE('',#6496,#6498,#4790,.T.);
#8303=EDGE_CURVE('',#6498,#6498,#1964,.T.);
#8304=EDGE_CURVE('',#6498,#6499,#4791,.T.);
#8305=EDGE_CURVE('',#6499,#6499,#1965,.T.);
#8306=EDGE_CURVE('',#6500,#6500,#1966,.T.);
#8307=EDGE_CURVE('',#6500,#6501,#4792,.T.);
#8308=EDGE_CURVE('',#6501,#6501,#1967,.T.);
#8309=EDGE_CURVE('',#6502,#6502,#1968,.T.);
#8310=EDGE_CURVE('',#6502,#6503,#4793,.T.);
#8311=EDGE_CURVE('',#6503,#6503,#1969,.T.);
#8312=EDGE_CURVE('',#6502,#6504,#4794,.T.);
#8313=EDGE_CURVE('',#6504,#6504,#1970,.T.);
#8314=EDGE_CURVE('',#6504,#6505,#4795,.T.);
#8315=EDGE_CURVE('',#6505,#6505,#1971,.T.);
#8316=EDGE_CURVE('',#6506,#6506,#1972,.T.);
#8317=EDGE_CURVE('',#6506,#6507,#4796,.T.);
#8318=EDGE_CURVE('',#6507,#6507,#1973,.T.);
#8319=EDGE_CURVE('',#6508,#6508,#1974,.T.);
#8320=EDGE_CURVE('',#6508,#6509,#4797,.T.);
#8321=EDGE_CURVE('',#6509,#6509,#1975,.T.);
#8322=EDGE_CURVE('',#6508,#6510,#4798,.T.);
#8323=EDGE_CURVE('',#6510,#6510,#1976,.T.);
#8324=EDGE_CURVE('',#6510,#6463,#4799,.T.);
#8325=EDGE_CURVE('',#6511,#6511,#1977,.T.);
#8326=EDGE_CURVE('',#6511,#6512,#4800,.T.);
#8327=EDGE_CURVE('',#6512,#6512,#1978,.T.);
#8328=EDGE_CURVE('',#6511,#6513,#4801,.T.);
#8329=EDGE_CURVE('',#6513,#6513,#1979,.T.);
#8330=EDGE_CURVE('',#6513,#6483,#4802,.T.);
#8331=EDGE_CURVE('',#6514,#6514,#1980,.T.);
#8332=EDGE_CURVE('',#6514,#6515,#4803,.T.);
#8333=EDGE_CURVE('',#6515,#6515,#1981,.T.);
#8334=EDGE_CURVE('',#6514,#6516,#4804,.T.);
#8335=EDGE_CURVE('',#6516,#6516,#1982,.T.);
#8336=EDGE_CURVE('',#6516,#6482,#4805,.T.);
#8337=EDGE_CURVE('',#6517,#6517,#1983,.T.);
#8338=EDGE_CURVE('',#6517,#6518,#4806,.T.);
#8339=EDGE_CURVE('',#6518,#6518,#1984,.T.);
#8340=EDGE_CURVE('',#6517,#6519,#4807,.T.);
#8341=EDGE_CURVE('',#6519,#6519,#1985,.T.);
#8342=EDGE_CURVE('',#6519,#6481,#4808,.T.);
#8343=EDGE_CURVE('',#6520,#6521,#4809,.T.);
#8344=EDGE_CURVE('',#6520,#6465,#4810,.T.);
#8345=EDGE_CURVE('',#6521,#6464,#4811,.T.);
#8346=EDGE_CURVE('',#6522,#6520,#4812,.T.);
#8347=EDGE_CURVE('',#6522,#6466,#4813,.T.);
#8348=EDGE_CURVE('',#6523,#6522,#4814,.T.);
#8349=EDGE_CURVE('',#6523,#6467,#4815,.T.);
#8350=EDGE_CURVE('',#6521,#6523,#4816,.T.);
#8351=EDGE_CURVE('',#6524,#6525,#4817,.T.);
#8352=EDGE_CURVE('',#6524,#6469,#4818,.T.);
#8353=EDGE_CURVE('',#6525,#6468,#4819,.T.);
#8354=EDGE_CURVE('',#6526,#6524,#4820,.T.);
#8355=EDGE_CURVE('',#6526,#6470,#4821,.T.);
#8356=EDGE_CURVE('',#6527,#6526,#4822,.T.);
#8357=EDGE_CURVE('',#6527,#6471,#4823,.T.);
#8358=EDGE_CURVE('',#6525,#6527,#4824,.T.);
#8359=EDGE_CURVE('',#6528,#6529,#4825,.T.);
#8360=EDGE_CURVE('',#6528,#6473,#4826,.T.);
#8361=EDGE_CURVE('',#6529,#6472,#4827,.T.);
#8362=EDGE_CURVE('',#6530,#6528,#4828,.T.);
#8363=EDGE_CURVE('',#6530,#6474,#4829,.T.);
#8364=EDGE_CURVE('',#6531,#6530,#4830,.T.);
#8365=EDGE_CURVE('',#6531,#6475,#4831,.T.);
#8366=EDGE_CURVE('',#6529,#6531,#4832,.T.);
#8367=EDGE_CURVE('',#6532,#6533,#4833,.T.);
#8368=EDGE_CURVE('',#6532,#6477,#4834,.T.);
#8369=EDGE_CURVE('',#6533,#6476,#4835,.T.);
#8370=EDGE_CURVE('',#6534,#6532,#4836,.T.);
#8371=EDGE_CURVE('',#6534,#6478,#4837,.T.);
#8372=EDGE_CURVE('',#6535,#6534,#4838,.T.);
#8373=EDGE_CURVE('',#6535,#6479,#4839,.T.);
#8374=EDGE_CURVE('',#6533,#6535,#4840,.T.);
#8375=EDGE_CURVE('',#6536,#6536,#1986,.T.);
#8376=EDGE_CURVE('',#6536,#6537,#4841,.T.);
#8377=EDGE_CURVE('',#6537,#6537,#1987,.T.);
#8378=EDGE_CURVE('',#6480,#6538,#4842,.T.);
#8379=EDGE_CURVE('',#6538,#6538,#1988,.T.);
#8380=EDGE_CURVE('',#6539,#6447,#4843,.T.);
#8381=EDGE_CURVE('',#6462,#6539,#4844,.T.);
#8382=EDGE_CURVE('',#6540,#6449,#4845,.T.);
#8383=EDGE_CURVE('',#6539,#6540,#4846,.T.);
#8384=EDGE_CURVE('',#6541,#6451,#4847,.T.);
#8385=EDGE_CURVE('',#6540,#6541,#4848,.T.);
#8386=EDGE_CURVE('',#6541,#6459,#4849,.T.);
#11207=ORIENTED_EDGE('',*,*,#8225,.T.);
#11208=ORIENTED_EDGE('',*,*,#8226,.T.);
#11209=ORIENTED_EDGE('',*,*,#8227,.T.);
#11210=ORIENTED_EDGE('',*,*,#8228,.F.);
#11211=ORIENTED_EDGE('',*,*,#8229,.T.);
#11212=ORIENTED_EDGE('',*,*,#8230,.T.);
#11213=ORIENTED_EDGE('',*,*,#8231,.T.);
#11214=ORIENTED_EDGE('',*,*,#8226,.F.);
#11215=ORIENTED_EDGE('',*,*,#8232,.T.);
#11216=ORIENTED_EDGE('',*,*,#8233,.T.);
#11217=ORIENTED_EDGE('',*,*,#8234,.T.);
#11218=ORIENTED_EDGE('',*,*,#8230,.F.);
#11219=ORIENTED_EDGE('',*,*,#8235,.T.);
#11220=ORIENTED_EDGE('',*,*,#8236,.T.);
#11221=ORIENTED_EDGE('',*,*,#8237,.T.);
#11222=ORIENTED_EDGE('',*,*,#8233,.F.);
#11223=ORIENTED_EDGE('',*,*,#8238,.T.);
#11224=ORIENTED_EDGE('',*,*,#8239,.T.);
#11225=ORIENTED_EDGE('',*,*,#8240,.T.);
#11226=ORIENTED_EDGE('',*,*,#8236,.F.);
#11227=ORIENTED_EDGE('',*,*,#8241,.T.);
#11228=ORIENTED_EDGE('',*,*,#8239,.F.);
#11229=ORIENTED_EDGE('',*,*,#8242,.T.);
#11230=ORIENTED_EDGE('',*,*,#8243,.T.);
#11231=ORIENTED_EDGE('',*,*,#8244,.T.);
#11232=ORIENTED_EDGE('',*,*,#8243,.F.);
#11233=ORIENTED_EDGE('',*,*,#8245,.T.);
#11234=ORIENTED_EDGE('',*,*,#8246,.T.);
#11235=ORIENTED_EDGE('',*,*,#8247,.T.);
#11236=ORIENTED_EDGE('',*,*,#8246,.F.);
#11237=ORIENTED_EDGE('',*,*,#8248,.T.);
#11238=ORIENTED_EDGE('',*,*,#8228,.T.);
#11239=ORIENTED_EDGE('',*,*,#8241,.F.);
#11240=ORIENTED_EDGE('',*,*,#8249,.F.);
#11241=ORIENTED_EDGE('',*,*,#8250,.F.);
#11242=ORIENTED_EDGE('',*,*,#8251,.T.);
#11243=ORIENTED_EDGE('',*,*,#8244,.F.);
#11244=ORIENTED_EDGE('',*,*,#8252,.F.);
#11245=ORIENTED_EDGE('',*,*,#8253,.F.);
#11246=ORIENTED_EDGE('',*,*,#8249,.T.);
#11247=ORIENTED_EDGE('',*,*,#8247,.F.);
#11248=ORIENTED_EDGE('',*,*,#8254,.F.);
#11249=ORIENTED_EDGE('',*,*,#8255,.F.);
#11250=ORIENTED_EDGE('',*,*,#8252,.T.);
#11251=ORIENTED_EDGE('',*,*,#8227,.F.);
#11252=ORIENTED_EDGE('',*,*,#8256,.F.);
#11253=ORIENTED_EDGE('',*,*,#8257,.F.);
#11254=ORIENTED_EDGE('',*,*,#8254,.T.);
#11255=ORIENTED_EDGE('',*,*,#8225,.F.);
#11256=ORIENTED_EDGE('',*,*,#8248,.F.);
#11257=ORIENTED_EDGE('',*,*,#8245,.F.);
#11258=ORIENTED_EDGE('',*,*,#8242,.F.);
#11259=ORIENTED_EDGE('',*,*,#8238,.F.);
#11260=ORIENTED_EDGE('',*,*,#8235,.F.);
#11261=ORIENTED_EDGE('',*,*,#8232,.F.);
#11262=ORIENTED_EDGE('',*,*,#8229,.F.);
#11263=ORIENTED_EDGE('',*,*,#8258,.T.);
#11264=ORIENTED_EDGE('',*,*,#8259,.T.);
#11265=ORIENTED_EDGE('',*,*,#8260,.T.);
#11266=ORIENTED_EDGE('',*,*,#8261,.T.);
#11267=ORIENTED_EDGE('',*,*,#8262,.T.);
#11268=ORIENTED_EDGE('',*,*,#8263,.T.);
#11269=ORIENTED_EDGE('',*,*,#8264,.T.);
#11270=ORIENTED_EDGE('',*,*,#8265,.T.);
#11271=ORIENTED_EDGE('',*,*,#8266,.T.);
#11272=ORIENTED_EDGE('',*,*,#8267,.T.);
#11273=ORIENTED_EDGE('',*,*,#8268,.T.);
#11274=ORIENTED_EDGE('',*,*,#8269,.T.);
#11275=ORIENTED_EDGE('',*,*,#8270,.T.);
#11276=ORIENTED_EDGE('',*,*,#8271,.T.);
#11277=ORIENTED_EDGE('',*,*,#8272,.T.);
#11278=ORIENTED_EDGE('',*,*,#8273,.T.);
#11279=ORIENTED_EDGE('',*,*,#8274,.T.);
#11280=ORIENTED_EDGE('',*,*,#8275,.T.);
#11281=ORIENTED_EDGE('',*,*,#8276,.T.);
#11282=ORIENTED_EDGE('',*,*,#8277,.T.);
#11283=ORIENTED_EDGE('',*,*,#8278,.T.);
#11284=ORIENTED_EDGE('',*,*,#8279,.T.);
#11285=ORIENTED_EDGE('',*,*,#8280,.T.);
#11286=ORIENTED_EDGE('',*,*,#8281,.F.);
#11287=ORIENTED_EDGE('',*,*,#8280,.F.);
#11288=ORIENTED_EDGE('',*,*,#8279,.F.);
#11289=ORIENTED_EDGE('',*,*,#8282,.T.);
#11290=ORIENTED_EDGE('',*,*,#8283,.T.);
#11291=ORIENTED_EDGE('',*,*,#8282,.F.);
#11292=ORIENTED_EDGE('',*,*,#8283,.F.);
#11293=ORIENTED_EDGE('',*,*,#8284,.T.);
#11294=ORIENTED_EDGE('',*,*,#8285,.T.);
#11295=ORIENTED_EDGE('',*,*,#8284,.F.);
#11296=ORIENTED_EDGE('',*,*,#8286,.T.);
#11297=ORIENTED_EDGE('',*,*,#8285,.F.);
#11298=ORIENTED_EDGE('',*,*,#8286,.F.);
#11299=ORIENTED_EDGE('',*,*,#8287,.T.);
#11300=ORIENTED_EDGE('',*,*,#8288,.F.);
#11301=ORIENTED_EDGE('',*,*,#8287,.F.);
#11302=ORIENTED_EDGE('',*,*,#8289,.T.);
#11303=ORIENTED_EDGE('',*,*,#8290,.T.);
#11304=ORIENTED_EDGE('',*,*,#8291,.F.);
#11305=ORIENTED_EDGE('',*,*,#8290,.F.);
#11306=ORIENTED_EDGE('',*,*,#8289,.F.);
#11307=ORIENTED_EDGE('',*,*,#8292,.T.);
#11308=ORIENTED_EDGE('',*,*,#8293,.T.);
#11309=ORIENTED_EDGE('',*,*,#8292,.F.);
#11310=ORIENTED_EDGE('',*,*,#8293,.F.);
#11311=ORIENTED_EDGE('',*,*,#8294,.T.);
#11312=ORIENTED_EDGE('',*,*,#8295,.T.);
#11313=ORIENTED_EDGE('',*,*,#8294,.F.);
#11314=ORIENTED_EDGE('',*,*,#8296,.T.);
#11315=ORIENTED_EDGE('',*,*,#8295,.F.);
#11316=ORIENTED_EDGE('',*,*,#8296,.F.);
#11317=ORIENTED_EDGE('',*,*,#8297,.T.);
#11318=ORIENTED_EDGE('',*,*,#8298,.F.);
#11319=ORIENTED_EDGE('',*,*,#8297,.F.);
#11320=ORIENTED_EDGE('',*,*,#8299,.T.);
#11321=ORIENTED_EDGE('',*,*,#8300,.T.);
#11322=ORIENTED_EDGE('',*,*,#8301,.F.);
#11323=ORIENTED_EDGE('',*,*,#8300,.F.);
#11324=ORIENTED_EDGE('',*,*,#8299,.F.);
#11325=ORIENTED_EDGE('',*,*,#8302,.T.);
#11326=ORIENTED_EDGE('',*,*,#8303,.T.);
#11327=ORIENTED_EDGE('',*,*,#8302,.F.);
#11328=ORIENTED_EDGE('',*,*,#8303,.F.);
#11329=ORIENTED_EDGE('',*,*,#8304,.T.);
#11330=ORIENTED_EDGE('',*,*,#8305,.T.);
#11331=ORIENTED_EDGE('',*,*,#8304,.F.);
#11332=ORIENTED_EDGE('',*,*,#8306,.T.);
#11333=ORIENTED_EDGE('',*,*,#8305,.F.);
#11334=ORIENTED_EDGE('',*,*,#8306,.F.);
#11335=ORIENTED_EDGE('',*,*,#8307,.T.);
#11336=ORIENTED_EDGE('',*,*,#8308,.F.);
#11337=ORIENTED_EDGE('',*,*,#8307,.F.);
#11338=ORIENTED_EDGE('',*,*,#8309,.T.);
#11339=ORIENTED_EDGE('',*,*,#8310,.T.);
#11340=ORIENTED_EDGE('',*,*,#8311,.F.);
#11341=ORIENTED_EDGE('',*,*,#8310,.F.);
#11342=ORIENTED_EDGE('',*,*,#8309,.F.);
#11343=ORIENTED_EDGE('',*,*,#8312,.T.);
#11344=ORIENTED_EDGE('',*,*,#8313,.T.);
#11345=ORIENTED_EDGE('',*,*,#8312,.F.);
#11346=ORIENTED_EDGE('',*,*,#8313,.F.);
#11347=ORIENTED_EDGE('',*,*,#8314,.T.);
#11348=ORIENTED_EDGE('',*,*,#8315,.T.);
#11349=ORIENTED_EDGE('',*,*,#8314,.F.);
#11350=ORIENTED_EDGE('',*,*,#8316,.T.);
#11351=ORIENTED_EDGE('',*,*,#8315,.F.);
#11352=ORIENTED_EDGE('',*,*,#8316,.F.);
#11353=ORIENTED_EDGE('',*,*,#8317,.T.);
#11354=ORIENTED_EDGE('',*,*,#8318,.F.);
#11355=ORIENTED_EDGE('',*,*,#8317,.F.);
#11356=ORIENTED_EDGE('',*,*,#8319,.T.);
#11357=ORIENTED_EDGE('',*,*,#8320,.T.);
#11358=ORIENTED_EDGE('',*,*,#8321,.F.);
#11359=ORIENTED_EDGE('',*,*,#8320,.F.);
#11360=ORIENTED_EDGE('',*,*,#8319,.F.);
#11361=ORIENTED_EDGE('',*,*,#8322,.T.);
#11362=ORIENTED_EDGE('',*,*,#8323,.T.);
#11363=ORIENTED_EDGE('',*,*,#8322,.F.);
#11364=ORIENTED_EDGE('',*,*,#8323,.F.);
#11365=ORIENTED_EDGE('',*,*,#8324,.T.);
#11366=ORIENTED_EDGE('',*,*,#8258,.F.);
#11367=ORIENTED_EDGE('',*,*,#8324,.F.);
#11368=ORIENTED_EDGE('',*,*,#8325,.T.);
#11369=ORIENTED_EDGE('',*,*,#8326,.T.);
#11370=ORIENTED_EDGE('',*,*,#8327,.F.);
#11371=ORIENTED_EDGE('',*,*,#8326,.F.);
#11372=ORIENTED_EDGE('',*,*,#8325,.F.);
#11373=ORIENTED_EDGE('',*,*,#8328,.T.);
#11374=ORIENTED_EDGE('',*,*,#8329,.T.);
#11375=ORIENTED_EDGE('',*,*,#8328,.F.);
#11376=ORIENTED_EDGE('',*,*,#8329,.F.);
#11377=ORIENTED_EDGE('',*,*,#8330,.T.);
#11378=ORIENTED_EDGE('',*,*,#8278,.F.);
#11379=ORIENTED_EDGE('',*,*,#8330,.F.);
#11380=ORIENTED_EDGE('',*,*,#8331,.T.);
#11381=ORIENTED_EDGE('',*,*,#8332,.T.);
#11382=ORIENTED_EDGE('',*,*,#8333,.F.);
#11383=ORIENTED_EDGE('',*,*,#8332,.F.);
#11384=ORIENTED_EDGE('',*,*,#8331,.F.);
#11385=ORIENTED_EDGE('',*,*,#8334,.T.);
#11386=ORIENTED_EDGE('',*,*,#8335,.T.);
#11387=ORIENTED_EDGE('',*,*,#8334,.F.);
#11388=ORIENTED_EDGE('',*,*,#8335,.F.);
#11389=ORIENTED_EDGE('',*,*,#8336,.T.);
#11390=ORIENTED_EDGE('',*,*,#8277,.F.);
#11391=ORIENTED_EDGE('',*,*,#8336,.F.);
#11392=ORIENTED_EDGE('',*,*,#8337,.T.);
#11393=ORIENTED_EDGE('',*,*,#8338,.T.);
#11394=ORIENTED_EDGE('',*,*,#8339,.F.);
#11395=ORIENTED_EDGE('',*,*,#8338,.F.);
#11396=ORIENTED_EDGE('',*,*,#8337,.F.);
#11397=ORIENTED_EDGE('',*,*,#8340,.T.);
#11398=ORIENTED_EDGE('',*,*,#8341,.T.);
#11399=ORIENTED_EDGE('',*,*,#8340,.F.);
#11400=ORIENTED_EDGE('',*,*,#8341,.F.);
#11401=ORIENTED_EDGE('',*,*,#8342,.T.);
#11402=ORIENTED_EDGE('',*,*,#8276,.F.);
#11403=ORIENTED_EDGE('',*,*,#8342,.F.);
#11404=ORIENTED_EDGE('',*,*,#8343,.F.);
#11405=ORIENTED_EDGE('',*,*,#8344,.T.);
#11406=ORIENTED_EDGE('',*,*,#8259,.F.);
#11407=ORIENTED_EDGE('',*,*,#8345,.F.);
#11408=ORIENTED_EDGE('',*,*,#8346,.F.);
#11409=ORIENTED_EDGE('',*,*,#8347,.T.);
#11410=ORIENTED_EDGE('',*,*,#8260,.F.);
#11411=ORIENTED_EDGE('',*,*,#8344,.F.);
#11412=ORIENTED_EDGE('',*,*,#8348,.F.);
#11413=ORIENTED_EDGE('',*,*,#8349,.T.);
#11414=ORIENTED_EDGE('',*,*,#8261,.F.);
#11415=ORIENTED_EDGE('',*,*,#8347,.F.);
#11416=ORIENTED_EDGE('',*,*,#8350,.F.);
#11417=ORIENTED_EDGE('',*,*,#8345,.T.);
#11418=ORIENTED_EDGE('',*,*,#8262,.F.);
#11419=ORIENTED_EDGE('',*,*,#8349,.F.);
#11420=ORIENTED_EDGE('',*,*,#8351,.F.);
#11421=ORIENTED_EDGE('',*,*,#8352,.T.);
#11422=ORIENTED_EDGE('',*,*,#8263,.F.);
#11423=ORIENTED_EDGE('',*,*,#8353,.F.);
#11424=ORIENTED_EDGE('',*,*,#8354,.F.);
#11425=ORIENTED_EDGE('',*,*,#8355,.T.);
#11426=ORIENTED_EDGE('',*,*,#8264,.F.);
#11427=ORIENTED_EDGE('',*,*,#8352,.F.);
#11428=ORIENTED_EDGE('',*,*,#8356,.F.);
#11429=ORIENTED_EDGE('',*,*,#8357,.T.);
#11430=ORIENTED_EDGE('',*,*,#8265,.F.);
#11431=ORIENTED_EDGE('',*,*,#8355,.F.);
#11432=ORIENTED_EDGE('',*,*,#8358,.F.);
#11433=ORIENTED_EDGE('',*,*,#8353,.T.);
#11434=ORIENTED_EDGE('',*,*,#8266,.F.);
#11435=ORIENTED_EDGE('',*,*,#8357,.F.);
#11436=ORIENTED_EDGE('',*,*,#8359,.F.);
#11437=ORIENTED_EDGE('',*,*,#8360,.T.);
#11438=ORIENTED_EDGE('',*,*,#8267,.F.);
#11439=ORIENTED_EDGE('',*,*,#8361,.F.);
#11440=ORIENTED_EDGE('',*,*,#8362,.F.);
#11441=ORIENTED_EDGE('',*,*,#8363,.T.);
#11442=ORIENTED_EDGE('',*,*,#8268,.F.);
#11443=ORIENTED_EDGE('',*,*,#8360,.F.);
#11444=ORIENTED_EDGE('',*,*,#8364,.F.);
#11445=ORIENTED_EDGE('',*,*,#8365,.T.);
#11446=ORIENTED_EDGE('',*,*,#8269,.F.);
#11447=ORIENTED_EDGE('',*,*,#8363,.F.);
#11448=ORIENTED_EDGE('',*,*,#8366,.F.);
#11449=ORIENTED_EDGE('',*,*,#8361,.T.);
#11450=ORIENTED_EDGE('',*,*,#8270,.F.);
#11451=ORIENTED_EDGE('',*,*,#8365,.F.);
#11452=ORIENTED_EDGE('',*,*,#8367,.F.);
#11453=ORIENTED_EDGE('',*,*,#8368,.T.);
#11454=ORIENTED_EDGE('',*,*,#8271,.F.);
#11455=ORIENTED_EDGE('',*,*,#8369,.F.);
#11456=ORIENTED_EDGE('',*,*,#8370,.F.);
#11457=ORIENTED_EDGE('',*,*,#8371,.T.);
#11458=ORIENTED_EDGE('',*,*,#8272,.F.);
#11459=ORIENTED_EDGE('',*,*,#8368,.F.);
#11460=ORIENTED_EDGE('',*,*,#8372,.F.);
#11461=ORIENTED_EDGE('',*,*,#8373,.T.);
#11462=ORIENTED_EDGE('',*,*,#8273,.F.);
#11463=ORIENTED_EDGE('',*,*,#8371,.F.);
#11464=ORIENTED_EDGE('',*,*,#8374,.F.);
#11465=ORIENTED_EDGE('',*,*,#8369,.T.);
#11466=ORIENTED_EDGE('',*,*,#8274,.F.);
#11467=ORIENTED_EDGE('',*,*,#8373,.F.);
#11468=ORIENTED_EDGE('',*,*,#8375,.F.);
#11469=ORIENTED_EDGE('',*,*,#8376,.T.);
#11470=ORIENTED_EDGE('',*,*,#8377,.F.);
#11471=ORIENTED_EDGE('',*,*,#8376,.F.);
#11472=ORIENTED_EDGE('',*,*,#8275,.F.);
#11473=ORIENTED_EDGE('',*,*,#8378,.T.);
#11474=ORIENTED_EDGE('',*,*,#8379,.T.);
#11475=ORIENTED_EDGE('',*,*,#8378,.F.);
#11476=ORIENTED_EDGE('',*,*,#8379,.F.);
#11477=ORIENTED_EDGE('',*,*,#8288,.T.);
#11478=ORIENTED_EDGE('',*,*,#8298,.T.);
#11479=ORIENTED_EDGE('',*,*,#8308,.T.);
#11480=ORIENTED_EDGE('',*,*,#8318,.T.);
#11481=ORIENTED_EDGE('',*,*,#8377,.T.);
#11482=ORIENTED_EDGE('',*,*,#8231,.F.);
#11483=ORIENTED_EDGE('',*,*,#8380,.F.);
#11484=ORIENTED_EDGE('',*,*,#8381,.F.);
#11485=ORIENTED_EDGE('',*,*,#8256,.T.);
#11486=ORIENTED_EDGE('',*,*,#8234,.F.);
#11487=ORIENTED_EDGE('',*,*,#8382,.F.);
#11488=ORIENTED_EDGE('',*,*,#8383,.F.);
#11489=ORIENTED_EDGE('',*,*,#8380,.T.);
#11490=ORIENTED_EDGE('',*,*,#8237,.F.);
#11491=ORIENTED_EDGE('',*,*,#8384,.F.);
#11492=ORIENTED_EDGE('',*,*,#8385,.F.);
#11493=ORIENTED_EDGE('',*,*,#8382,.T.);
#11494=ORIENTED_EDGE('',*,*,#8240,.F.);
#11495=ORIENTED_EDGE('',*,*,#8251,.F.);
#11496=ORIENTED_EDGE('',*,*,#8386,.F.);
#11497=ORIENTED_EDGE('',*,*,#8384,.T.);
#11498=ORIENTED_EDGE('',*,*,#8386,.T.);
#11499=ORIENTED_EDGE('',*,*,#8250,.T.);
#11500=ORIENTED_EDGE('',*,*,#8253,.T.);
#11501=ORIENTED_EDGE('',*,*,#8255,.T.);
#11502=ORIENTED_EDGE('',*,*,#8257,.T.);
#11503=ORIENTED_EDGE('',*,*,#8381,.T.);
#11504=ORIENTED_EDGE('',*,*,#8383,.T.);
#11505=ORIENTED_EDGE('',*,*,#8385,.T.);
#11506=ORIENTED_EDGE('',*,*,#8291,.T.);
#11507=ORIENTED_EDGE('',*,*,#8311,.T.);
#11508=ORIENTED_EDGE('',*,*,#8327,.T.);
#11509=ORIENTED_EDGE('',*,*,#8333,.T.);
#11510=ORIENTED_EDGE('',*,*,#8339,.T.);
#11511=ORIENTED_EDGE('',*,*,#8375,.T.);
#11512=ORIENTED_EDGE('',*,*,#8367,.T.);
#11513=ORIENTED_EDGE('',*,*,#8374,.T.);
#11514=ORIENTED_EDGE('',*,*,#8372,.T.);
#11515=ORIENTED_EDGE('',*,*,#8370,.T.);
#11516=ORIENTED_EDGE('',*,*,#8359,.T.);
#11517=ORIENTED_EDGE('',*,*,#8366,.T.);
#11518=ORIENTED_EDGE('',*,*,#8364,.T.);
#11519=ORIENTED_EDGE('',*,*,#8362,.T.);
#11520=ORIENTED_EDGE('',*,*,#8351,.T.);
#11521=ORIENTED_EDGE('',*,*,#8358,.T.);
#11522=ORIENTED_EDGE('',*,*,#8356,.T.);
#11523=ORIENTED_EDGE('',*,*,#8354,.T.);
#11524=ORIENTED_EDGE('',*,*,#8343,.T.);
#11525=ORIENTED_EDGE('',*,*,#8350,.T.);
#11526=ORIENTED_EDGE('',*,*,#8348,.T.);
#11527=ORIENTED_EDGE('',*,*,#8346,.T.);
#11528=ORIENTED_EDGE('',*,*,#8321,.T.);
#11529=ORIENTED_EDGE('',*,*,#8301,.T.);
#11530=ORIENTED_EDGE('',*,*,#8281,.T.);
#14603=PLANE('',#16306);
#14604=PLANE('',#16307);
#14605=PLANE('',#16308);
#14606=PLANE('',#16309);
#14607=PLANE('',#16310);
#14608=PLANE('',#16311);
#14609=PLANE('',#16312);
#14610=PLANE('',#16313);
#14611=PLANE('',#16314);
#14612=PLANE('',#16315);
#14613=PLANE('',#16316);
#14614=PLANE('',#16317);
#14615=PLANE('',#16318);
#14616=PLANE('',#16331);
#14617=PLANE('',#16342);
#14618=PLANE('',#16353);
#14619=PLANE('',#16364);
#14620=PLANE('',#16392);
#14621=PLANE('',#16393);
#14622=PLANE('',#16394);
#14623=PLANE('',#16395);
#14624=PLANE('',#16396);
#14625=PLANE('',#16397);
#14626=PLANE('',#16398);
#14627=PLANE('',#16399);
#14628=PLANE('',#16400);
#14629=PLANE('',#16401);
#14630=PLANE('',#16402);
#14631=PLANE('',#16403);
#14632=PLANE('',#16404);
#14633=PLANE('',#16405);
#14634=PLANE('',#16406);
#14635=PLANE('',#16407);
#14636=PLANE('',#16413);
#14637=PLANE('',#16414);
#14638=PLANE('',#16415);
#14639=PLANE('',#16416);
#14640=PLANE('',#16417);
#14641=PLANE('',#16418);
#15018=ADVANCED_FACE('',(#2662),#14603,.T.);
#15019=ADVANCED_FACE('',(#2663),#14604,.T.);
#15020=ADVANCED_FACE('',(#2664),#14605,.T.);
#15021=ADVANCED_FACE('',(#2665),#14606,.T.);
#15022=ADVANCED_FACE('',(#2666),#14607,.T.);
#15023=ADVANCED_FACE('',(#2667),#14608,.T.);
#15024=ADVANCED_FACE('',(#2668),#14609,.T.);
#15025=ADVANCED_FACE('',(#2669),#14610,.T.);
#15026=ADVANCED_FACE('',(#2670),#14611,.T.);
#15027=ADVANCED_FACE('',(#2671),#14612,.T.);
#15028=ADVANCED_FACE('',(#2672),#14613,.T.);
#15029=ADVANCED_FACE('',(#2673),#14614,.T.);
#15030=ADVANCED_FACE('',(#2674,#1668,#1669,#1670,#1671,#1672,#1673,#1674,
#1675,#1676),#14615,.T.);
#15031=ADVANCED_FACE('',(#2675),#1211,.F.);
#15032=ADVANCED_FACE('',(#2676),#1418,.F.);
#15033=ADVANCED_FACE('',(#2677),#1212,.F.);
#15034=ADVANCED_FACE('',(#2678,#1677),#14616,.F.);
#15035=ADVANCED_FACE('',(#2679),#1419,.F.);
#15036=ADVANCED_FACE('',(#2680),#1213,.F.);
#15037=ADVANCED_FACE('',(#2681),#1420,.F.);
#15038=ADVANCED_FACE('',(#2682),#1214,.F.);
#15039=ADVANCED_FACE('',(#2683,#1678),#14617,.F.);
#15040=ADVANCED_FACE('',(#2684),#1421,.F.);
#15041=ADVANCED_FACE('',(#2685),#1215,.F.);
#15042=ADVANCED_FACE('',(#2686),#1422,.F.);
#15043=ADVANCED_FACE('',(#2687),#1216,.F.);
#15044=ADVANCED_FACE('',(#2688,#1679),#14618,.F.);
#15045=ADVANCED_FACE('',(#2689),#1423,.F.);
#15046=ADVANCED_FACE('',(#2690),#1217,.F.);
#15047=ADVANCED_FACE('',(#2691),#1424,.F.);
#15048=ADVANCED_FACE('',(#2692),#1218,.F.);
#15049=ADVANCED_FACE('',(#2693,#1680),#14619,.F.);
#15050=ADVANCED_FACE('',(#2694),#1425,.F.);
#15051=ADVANCED_FACE('',(#2695),#1219,.F.);
#15052=ADVANCED_FACE('',(#2696),#1426,.F.);
#15053=ADVANCED_FACE('',(#2697),#1220,.F.);
#15054=ADVANCED_FACE('',(#2698),#1221,.F.);
#15055=ADVANCED_FACE('',(#2699),#1427,.F.);
#15056=ADVANCED_FACE('',(#2700),#1222,.F.);
#15057=ADVANCED_FACE('',(#2701),#1223,.F.);
#15058=ADVANCED_FACE('',(#2702),#1428,.F.);
#15059=ADVANCED_FACE('',(#2703),#1224,.F.);
#15060=ADVANCED_FACE('',(#2704),#1225,.F.);
#15061=ADVANCED_FACE('',(#2705),#1429,.F.);
#15062=ADVANCED_FACE('',(#2706),#1226,.F.);
#15063=ADVANCED_FACE('',(#2707),#14620,.F.);
#15064=ADVANCED_FACE('',(#2708),#14621,.F.);
#15065=ADVANCED_FACE('',(#2709),#14622,.F.);
#15066=ADVANCED_FACE('',(#2710),#14623,.F.);
#15067=ADVANCED_FACE('',(#2711),#14624,.F.);
#15068=ADVANCED_FACE('',(#2712),#14625,.F.);
#15069=ADVANCED_FACE('',(#2713),#14626,.F.);
#15070=ADVANCED_FACE('',(#2714),#14627,.F.);
#15071=ADVANCED_FACE('',(#2715),#14628,.F.);
#15072=ADVANCED_FACE('',(#2716),#14629,.F.);
#15073=ADVANCED_FACE('',(#2717),#14630,.F.);
#15074=ADVANCED_FACE('',(#2718),#14631,.F.);
#15075=ADVANCED_FACE('',(#2719),#14632,.F.);
#15076=ADVANCED_FACE('',(#2720),#14633,.F.);
#15077=ADVANCED_FACE('',(#2721),#14634,.F.);
#15078=ADVANCED_FACE('',(#2722),#14635,.F.);
#15079=ADVANCED_FACE('',(#2723),#1430,.F.);
#15080=ADVANCED_FACE('',(#2724),#1431,.F.);
#15081=ADVANCED_FACE('',(#2725,#1681,#1682,#1683,#1684,#1685),#14636,.F.);
#15082=ADVANCED_FACE('',(#2726),#14637,.T.);
#15083=ADVANCED_FACE('',(#2727),#14638,.T.);
#15084=ADVANCED_FACE('',(#2728),#14639,.T.);
#15085=ADVANCED_FACE('',(#2729),#14640,.T.);
#15086=ADVANCED_FACE('',(#2730,#1686,#1687,#1688,#1689,#1690,#1691,#1692,
#1693,#1694,#1695,#1696,#1697,#1698),#14641,.T.);
#15615=CLOSED_SHELL('',(#15018,#15019,#15020,#15021,#15022,#15023,#15024,
#15025,#15026,#15027,#15028,#15029,#15030,#15031,#15032,#15033,#15034,#15035,
#15036,#15037,#15038,#15039,#15040,#15041,#15042,#15043,#15044,#15045,#15046,
#15047,#15048,#15049,#15050,#15051,#15052,#15053,#15054,#15055,#15056,#15057,
#15058,#15059,#15060,#15061,#15062,#15063,#15064,#15065,#15066,#15067,#15068,
#15069,#15070,#15071,#15072,#15073,#15074,#15075,#15076,#15077,#15078,#15079,
#15080,#15081,#15082,#15083,#15084,#15085,#15086));
#16305=AXIS2_PLACEMENT_3D('',#22789,#18687,#18688);
#16306=AXIS2_PLACEMENT_3D('',#22790,#18689,#18690);
#16307=AXIS2_PLACEMENT_3D('',#22799,#18695,#18696);
#16308=AXIS2_PLACEMENT_3D('',#22805,#18700,#18701);
#16309=AXIS2_PLACEMENT_3D('',#22811,#18705,#18706);
#16310=AXIS2_PLACEMENT_3D('',#22817,#18710,#18711);
#16311=AXIS2_PLACEMENT_3D('',#22823,#18715,#18716);
#16312=AXIS2_PLACEMENT_3D('',#22829,#18720,#18721);
#16313=AXIS2_PLACEMENT_3D('',#22835,#18725,#18726);
#16314=AXIS2_PLACEMENT_3D('',#22838,#18729,#18730);
#16315=AXIS2_PLACEMENT_3D('',#22844,#18734,#18735);
#16316=AXIS2_PLACEMENT_3D('',#22848,#18738,#18739);
#16317=AXIS2_PLACEMENT_3D('',#22852,#18742,#18743);
#16318=AXIS2_PLACEMENT_3D('',#22856,#18746,#18747);
#16319=AXIS2_PLACEMENT_3D('',#22858,#18748,#18749);
#16320=AXIS2_PLACEMENT_3D('',#22892,#18766,#18767);
#16321=AXIS2_PLACEMENT_3D('',#22894,#18768,#18769);
#16322=AXIS2_PLACEMENT_3D('',#22896,#18770,#18771);
#16323=AXIS2_PLACEMENT_3D('',#22898,#18772,#18773);
#16324=AXIS2_PLACEMENT_3D('',#22899,#18774,#18775);
#16325=AXIS2_PLACEMENT_3D('',#22901,#18776,#18777);
#16326=AXIS2_PLACEMENT_3D('',#22904,#18779,#18780);
#16327=AXIS2_PLACEMENT_3D('',#22905,#18781,#18782);
#16328=AXIS2_PLACEMENT_3D('',#22908,#18784,#18785);
#16329=AXIS2_PLACEMENT_3D('',#22909,#18786,#18787);
#16330=AXIS2_PLACEMENT_3D('',#22912,#18789,#18790);
#16331=AXIS2_PLACEMENT_3D('',#22913,#18791,#18792);
#16332=AXIS2_PLACEMENT_3D('',#22915,#18793,#18794);
#16333=AXIS2_PLACEMENT_3D('',#22916,#18795,#18796);
#16334=AXIS2_PLACEMENT_3D('',#22919,#18798,#18799);
#16335=AXIS2_PLACEMENT_3D('',#22920,#18800,#18801);
#16336=AXIS2_PLACEMENT_3D('',#22922,#18802,#18803);
#16337=AXIS2_PLACEMENT_3D('',#22925,#18805,#18806);
#16338=AXIS2_PLACEMENT_3D('',#22926,#18807,#18808);
#16339=AXIS2_PLACEMENT_3D('',#22929,#18810,#18811);
#16340=AXIS2_PLACEMENT_3D('',#22930,#18812,#18813);
#16341=AXIS2_PLACEMENT_3D('',#22933,#18815,#18816);
#16342=AXIS2_PLACEMENT_3D('',#22934,#18817,#18818);
#16343=AXIS2_PLACEMENT_3D('',#22936,#18819,#18820);
#16344=AXIS2_PLACEMENT_3D('',#22937,#18821,#18822);
#16345=AXIS2_PLACEMENT_3D('',#22940,#18824,#18825);
#16346=AXIS2_PLACEMENT_3D('',#22941,#18826,#18827);
#16347=AXIS2_PLACEMENT_3D('',#22943,#18828,#18829);
#16348=AXIS2_PLACEMENT_3D('',#22946,#18831,#18832);
#16349=AXIS2_PLACEMENT_3D('',#22947,#18833,#18834);
#16350=AXIS2_PLACEMENT_3D('',#22950,#18836,#18837);
#16351=AXIS2_PLACEMENT_3D('',#22951,#18838,#18839);
#16352=AXIS2_PLACEMENT_3D('',#22954,#18841,#18842);
#16353=AXIS2_PLACEMENT_3D('',#22955,#18843,#18844);
#16354=AXIS2_PLACEMENT_3D('',#22957,#18845,#18846);
#16355=AXIS2_PLACEMENT_3D('',#22958,#18847,#18848);
#16356=AXIS2_PLACEMENT_3D('',#22961,#18850,#18851);
#16357=AXIS2_PLACEMENT_3D('',#22962,#18852,#18853);
#16358=AXIS2_PLACEMENT_3D('',#22964,#18854,#18855);
#16359=AXIS2_PLACEMENT_3D('',#22967,#18857,#18858);
#16360=AXIS2_PLACEMENT_3D('',#22968,#18859,#18860);
#16361=AXIS2_PLACEMENT_3D('',#22971,#18862,#18863);
#16362=AXIS2_PLACEMENT_3D('',#22972,#18864,#18865);
#16363=AXIS2_PLACEMENT_3D('',#22975,#18867,#18868);
#16364=AXIS2_PLACEMENT_3D('',#22976,#18869,#18870);
#16365=AXIS2_PLACEMENT_3D('',#22978,#18871,#18872);
#16366=AXIS2_PLACEMENT_3D('',#22979,#18873,#18874);
#16367=AXIS2_PLACEMENT_3D('',#22982,#18876,#18877);
#16368=AXIS2_PLACEMENT_3D('',#22983,#18878,#18879);
#16369=AXIS2_PLACEMENT_3D('',#22985,#18880,#18881);
#16370=AXIS2_PLACEMENT_3D('',#22988,#18883,#18884);
#16371=AXIS2_PLACEMENT_3D('',#22989,#18885,#18886);
#16372=AXIS2_PLACEMENT_3D('',#22992,#18888,#18889);
#16373=AXIS2_PLACEMENT_3D('',#22993,#18890,#18891);
#16374=AXIS2_PLACEMENT_3D('',#22995,#18893,#18894);
#16375=AXIS2_PLACEMENT_3D('',#22997,#18895,#18896);
#16376=AXIS2_PLACEMENT_3D('',#23000,#18898,#18899);
#16377=AXIS2_PLACEMENT_3D('',#23001,#18900,#18901);
#16378=AXIS2_PLACEMENT_3D('',#23004,#18903,#18904);
#16379=AXIS2_PLACEMENT_3D('',#23005,#18905,#18906);
#16380=AXIS2_PLACEMENT_3D('',#23007,#18908,#18909);
#16381=AXIS2_PLACEMENT_3D('',#23009,#18910,#18911);
#16382=AXIS2_PLACEMENT_3D('',#23012,#18913,#18914);
#16383=AXIS2_PLACEMENT_3D('',#23013,#18915,#18916);
#16384=AXIS2_PLACEMENT_3D('',#23016,#18918,#18919);
#16385=AXIS2_PLACEMENT_3D('',#23017,#18920,#18921);
#16386=AXIS2_PLACEMENT_3D('',#23019,#18923,#18924);
#16387=AXIS2_PLACEMENT_3D('',#23021,#18925,#18926);
#16388=AXIS2_PLACEMENT_3D('',#23024,#18928,#18929);
#16389=AXIS2_PLACEMENT_3D('',#23025,#18930,#18931);
#16390=AXIS2_PLACEMENT_3D('',#23028,#18933,#18934);
#16391=AXIS2_PLACEMENT_3D('',#23029,#18935,#18936);
#16392=AXIS2_PLACEMENT_3D('',#23031,#18938,#18939);
#16393=AXIS2_PLACEMENT_3D('',#23037,#18943,#18944);
#16394=AXIS2_PLACEMENT_3D('',#23041,#18947,#18948);
#16395=AXIS2_PLACEMENT_3D('',#23045,#18951,#18952);
#16396=AXIS2_PLACEMENT_3D('',#23047,#18954,#18955);
#16397=AXIS2_PLACEMENT_3D('',#23053,#18959,#18960);
#16398=AXIS2_PLACEMENT_3D('',#23057,#18963,#18964);
#16399=AXIS2_PLACEMENT_3D('',#23061,#18967,#18968);
#16400=AXIS2_PLACEMENT_3D('',#23063,#18970,#18971);
#16401=AXIS2_PLACEMENT_3D('',#23069,#18975,#18976);
#16402=AXIS2_PLACEMENT_3D('',#23073,#18979,#18980);
#16403=AXIS2_PLACEMENT_3D('',#23077,#18983,#18984);
#16404=AXIS2_PLACEMENT_3D('',#23079,#18986,#18987);
#16405=AXIS2_PLACEMENT_3D('',#23085,#18991,#18992);
#16406=AXIS2_PLACEMENT_3D('',#23089,#18995,#18996);
#16407=AXIS2_PLACEMENT_3D('',#23093,#18999,#19000);
#16408=AXIS2_PLACEMENT_3D('',#23095,#19002,#19003);
#16409=AXIS2_PLACEMENT_3D('',#23097,#19004,#19005);
#16410=AXIS2_PLACEMENT_3D('',#23100,#19007,#19008);
#16411=AXIS2_PLACEMENT_3D('',#23101,#19009,#19010);
#16412=AXIS2_PLACEMENT_3D('',#23104,#19012,#19013);
#16413=AXIS2_PLACEMENT_3D('',#23105,#19014,#19015);
#16414=AXIS2_PLACEMENT_3D('',#23106,#19016,#19017);
#16415=AXIS2_PLACEMENT_3D('',#23110,#19020,#19021);
#16416=AXIS2_PLACEMENT_3D('',#23114,#19024,#19025);
#16417=AXIS2_PLACEMENT_3D('',#23118,#19028,#19029);
#16418=AXIS2_PLACEMENT_3D('',#23120,#19031,#19032);
#18687=DIRECTION('axis',(0.,0.,1.));
#18688=DIRECTION('refdir',(1.,0.,0.));
#18689=DIRECTION('center_axis',(-0.707106781186548,0.5,0.5));
#18690=DIRECTION('ref_axis',(0.577350269189625,-1.05152891894174E-16,0.816496580927726));
#18691=DIRECTION('',(0.,-0.707106781186548,0.707106781186547));
#18692=DIRECTION('',(0.678598344545845,0.281084637714803,0.678598344545857));
#18693=DIRECTION('',(0.,0.707106781186548,-0.707106781186547));
#18694=DIRECTION('',(0.678598344545846,0.678598344545852,0.281084637714809));
#18695=DIRECTION('center_axis',(-0.707106781186554,0.,0.707106781186541));
#18696=DIRECTION('ref_axis',(0.707106781186541,0.,0.707106781186554));
#18697=DIRECTION('',(0.,-1.,0.));
#18698=DIRECTION('',(0.678598344545847,-0.281084637714792,0.678598344545859));
#18699=DIRECTION('',(0.,1.,0.));
#18700=DIRECTION('center_axis',(-0.707106781186544,-0.500000000000003,0.500000000000003));
#18701=DIRECTION('ref_axis',(0.57735026918963,1.66848612271393E-17,0.816496580927723));
#18702=DIRECTION('',(0.,-0.707106781186548,-0.707106781186547));
#18703=DIRECTION('',(0.678598344545849,-0.678598344545849,0.281084637714811));
#18704=DIRECTION('',(0.,0.707106781186548,0.707106781186547));
#18705=DIRECTION('center_axis',(-0.707106781186548,-0.707106781186548,0.));
#18706=DIRECTION('ref_axis',(0.,0.,1.));
#18707=DIRECTION('',(0.,0.,-1.));
#18708=DIRECTION('',(0.678598344545844,-0.678598344545844,-0.281084637714833));
#18709=DIRECTION('',(0.,0.,1.));
#18710=DIRECTION('center_axis',(-0.707106781186553,-0.499999999999996,-0.499999999999996));
#18711=DIRECTION('ref_axis',(-0.57735026918962,1.74145151191031E-16,0.81649658092773));
#18712=DIRECTION('',(0.,0.707106781186548,-0.707106781186548));
#18713=DIRECTION('',(0.678598344545843,-0.281084637714838,-0.678598344545843));
#18714=DIRECTION('',(0.,-0.707106781186548,0.707106781186548));
#18715=DIRECTION('center_axis',(-0.707106781186548,0.,-0.707106781186548));
#18716=DIRECTION('ref_axis',(-0.707106781186548,0.,0.707106781186548));
#18717=DIRECTION('',(0.,-1.,0.));
#18718=DIRECTION('',(0.,1.,0.));
#18719=DIRECTION('',(0.678598344545846,0.281084637714827,-0.678598344545846));
#18720=DIRECTION('center_axis',(-0.707106781186548,0.5,-0.5));
#18721=DIRECTION('ref_axis',(-0.577350269189625,1.05152891894174E-16,0.816496580927726));
#18722=DIRECTION('',(0.,-0.707106781186548,-0.707106781186548));
#18723=DIRECTION('',(0.,0.707106781186548,0.707106781186548));
#18724=DIRECTION('',(0.678598344545846,0.678598344545846,-0.281084637714827));
#18725=DIRECTION('center_axis',(-0.707106781186548,0.707106781186548,0.));
#18726=DIRECTION('ref_axis',(0.,0.,1.));
#18727=DIRECTION('',(0.,0.,-1.));
#18728=DIRECTION('',(0.,0.,1.));
#18729=DIRECTION('center_axis',(0.,0.,-1.));
#18730=DIRECTION('ref_axis',(0.,-1.,0.));
#18731=DIRECTION('',(-1.,0.,0.));
#18732=DIRECTION('',(0.,1.,0.));
#18733=DIRECTION('',(-1.,0.,0.));
#18734=DIRECTION('center_axis',(0.,0.707106781186548,-0.707106781186548));
#18735=DIRECTION('ref_axis',(0.,-0.707106781186548,-0.707106781186548));
#18736=DIRECTION('',(-1.,0.,0.));
#18737=DIRECTION('',(0.,0.707106781186548,0.707106781186548));
#18738=DIRECTION('center_axis',(0.,1.,0.));
#18739=DIRECTION('ref_axis',(0.,0.,-1.));
#18740=DIRECTION('',(-1.,0.,0.));
#18741=DIRECTION('',(0.,0.,1.));
#18742=DIRECTION('center_axis',(0.,0.707106781186547,0.707106781186548));
#18743=DIRECTION('ref_axis',(0.,0.707106781186548,-0.707106781186547));
#18744=DIRECTION('',(-1.,0.,0.));
#18745=DIRECTION('',(0.,-0.707106781186548,0.707106781186547));
#18746=DIRECTION('center_axis',(-1.,0.,0.));
#18747=DIRECTION('ref_axis',(0.,0.,1.));
#18748=DIRECTION('center_axis',(1.,0.,0.));
#18749=DIRECTION('ref_axis',(0.,-1.,0.));
#18750=DIRECTION('',(0.,1.,0.));
#18751=DIRECTION('',(0.,0.,1.));
#18752=DIRECTION('',(0.,-1.,0.));
#18753=DIRECTION('',(0.,0.,-1.));
#18754=DIRECTION('',(0.,1.,0.));
#18755=DIRECTION('',(0.,0.,1.));
#18756=DIRECTION('',(0.,-1.,0.));
#18757=DIRECTION('',(0.,0.,-1.));
#18758=DIRECTION('',(0.,1.,0.));
#18759=DIRECTION('',(0.,0.,1.));
#18760=DIRECTION('',(0.,-1.,0.));
#18761=DIRECTION('',(0.,0.,-1.));
#18762=DIRECTION('',(0.,1.,0.));
#18763=DIRECTION('',(0.,0.,1.));
#18764=DIRECTION('',(0.,-1.,0.));
#18765=DIRECTION('',(0.,0.,-1.));
#18766=DIRECTION('center_axis',(1.,0.,0.));
#18767=DIRECTION('ref_axis',(0.,0.,-1.));
#18768=DIRECTION('center_axis',(1.,0.,0.));
#18769=DIRECTION('ref_axis',(0.,-1.,0.));
#18770=DIRECTION('center_axis',(1.,0.,0.));
#18771=DIRECTION('ref_axis',(0.,-1.,0.));
#18772=DIRECTION('center_axis',(1.,0.,0.));
#18773=DIRECTION('ref_axis',(0.,-1.,0.));
#18774=DIRECTION('center_axis',(1.,0.,0.));
#18775=DIRECTION('ref_axis',(0.,-1.,0.));
#18776=DIRECTION('center_axis',(-1.,0.,0.));
#18777=DIRECTION('ref_axis',(0.,0.,1.));
#18778=DIRECTION('',(0.948683298050512,0.316227766016844,3.87267321454047E-17));
#18779=DIRECTION('center_axis',(-1.,0.,0.));
#18780=DIRECTION('ref_axis',(0.,-1.,0.));
#18781=DIRECTION('center_axis',(-1.,0.,0.));
#18782=DIRECTION('ref_axis',(0.,-1.,0.));
#18783=DIRECTION('',(-1.,0.,0.));
#18784=DIRECTION('center_axis',(-1.,0.,0.));
#18785=DIRECTION('ref_axis',(0.,0.,1.));
#18786=DIRECTION('center_axis',(-1.,0.,0.));
#18787=DIRECTION('ref_axis',(0.,-1.,0.));
#18788=DIRECTION('',(-0.707106781186535,0.70710678118656,-8.65956056235509E-17));
#18789=DIRECTION('center_axis',(-1.,0.,0.));
#18790=DIRECTION('ref_axis',(0.,0.,1.));
#18791=DIRECTION('center_axis',(1.,0.,0.));
#18792=DIRECTION('ref_axis',(0.,0.,-1.));
#18793=DIRECTION('center_axis',(-1.,0.,0.));
#18794=DIRECTION('ref_axis',(0.,0.,1.));
#18795=DIRECTION('center_axis',(-1.,0.,0.));
#18796=DIRECTION('ref_axis',(0.,-1.,0.));
#18797=DIRECTION('',(-1.,0.,0.));
#18798=DIRECTION('center_axis',(1.,0.,0.));
#18799=DIRECTION('ref_axis',(0.,-1.,0.));
#18800=DIRECTION('center_axis',(1.,0.,0.));
#18801=DIRECTION('ref_axis',(0.,-1.,0.));
#18802=DIRECTION('center_axis',(-1.,0.,0.));
#18803=DIRECTION('ref_axis',(0.,0.,1.));
#18804=DIRECTION('',(0.948683298050513,0.31622776601684,3.87267321454041E-17));
#18805=DIRECTION('center_axis',(-1.,0.,0.));
#18806=DIRECTION('ref_axis',(0.,-1.,0.));
#18807=DIRECTION('center_axis',(-1.,0.,0.));
#18808=DIRECTION('ref_axis',(0.,-1.,0.));
#18809=DIRECTION('',(-1.,0.,0.));
#18810=DIRECTION('center_axis',(-1.,0.,0.));
#18811=DIRECTION('ref_axis',(0.,0.,1.));
#18812=DIRECTION('center_axis',(-1.,0.,0.));
#18813=DIRECTION('ref_axis',(0.,-1.,0.));
#18814=DIRECTION('',(-0.707106781186541,0.707106781186554,-8.65956056235501E-17));
#18815=DIRECTION('center_axis',(-1.,0.,0.));
#18816=DIRECTION('ref_axis',(0.,0.,1.));
#18817=DIRECTION('center_axis',(1.,0.,0.));
#18818=DIRECTION('ref_axis',(0.,0.,-1.));
#18819=DIRECTION('center_axis',(-1.,0.,0.));
#18820=DIRECTION('ref_axis',(0.,0.,1.));
#18821=DIRECTION('center_axis',(-1.,0.,0.));
#18822=DIRECTION('ref_axis',(0.,-1.,0.));
#18823=DIRECTION('',(-1.,0.,0.));
#18824=DIRECTION('center_axis',(1.,0.,0.));
#18825=DIRECTION('ref_axis',(0.,-1.,0.));
#18826=DIRECTION('center_axis',(1.,0.,0.));
#18827=DIRECTION('ref_axis',(0.,-1.,0.));
#18828=DIRECTION('center_axis',(-1.,0.,0.));
#18829=DIRECTION('ref_axis',(0.,0.,1.));
#18830=DIRECTION('',(0.948683298050512,0.316227766016844,3.87267321454047E-17));
#18831=DIRECTION('center_axis',(-1.,0.,0.));
#18832=DIRECTION('ref_axis',(0.,-1.,0.));
#18833=DIRECTION('center_axis',(-1.,0.,0.));
#18834=DIRECTION('ref_axis',(0.,-1.,0.));
#18835=DIRECTION('',(-1.,0.,0.));
#18836=DIRECTION('center_axis',(-1.,0.,0.));
#18837=DIRECTION('ref_axis',(0.,0.,1.));
#18838=DIRECTION('center_axis',(-1.,0.,0.));
#18839=DIRECTION('ref_axis',(0.,-1.,0.));
#18840=DIRECTION('',(-0.707106781186535,0.70710678118656,-8.65956056235509E-17));
#18841=DIRECTION('center_axis',(-1.,0.,0.));
#18842=DIRECTION('ref_axis',(0.,0.,1.));
#18843=DIRECTION('center_axis',(1.,0.,0.));
#18844=DIRECTION('ref_axis',(0.,0.,-1.));
#18845=DIRECTION('center_axis',(-1.,0.,0.));
#18846=DIRECTION('ref_axis',(0.,0.,1.));
#18847=DIRECTION('center_axis',(-1.,0.,0.));
#18848=DIRECTION('ref_axis',(0.,-1.,0.));
#18849=DIRECTION('',(-1.,0.,0.));
#18850=DIRECTION('center_axis',(1.,0.,0.));
#18851=DIRECTION('ref_axis',(0.,-1.,0.));
#18852=DIRECTION('center_axis',(1.,0.,0.));
#18853=DIRECTION('ref_axis',(0.,-1.,0.));
#18854=DIRECTION('center_axis',(-1.,0.,0.));
#18855=DIRECTION('ref_axis',(0.,0.,1.));
#18856=DIRECTION('',(0.948683298050513,0.31622776601684,3.87267321454041E-17));
#18857=DIRECTION('center_axis',(-1.,0.,0.));
#18858=DIRECTION('ref_axis',(0.,-1.,0.));
#18859=DIRECTION('center_axis',(-1.,0.,0.));
#18860=DIRECTION('ref_axis',(0.,-1.,0.));
#18861=DIRECTION('',(-1.,0.,0.));
#18862=DIRECTION('center_axis',(-1.,0.,0.));
#18863=DIRECTION('ref_axis',(0.,0.,1.));
#18864=DIRECTION('center_axis',(-1.,0.,0.));
#18865=DIRECTION('ref_axis',(0.,-1.,0.));
#18866=DIRECTION('',(-0.707106781186541,0.707106781186554,-8.65956056235501E-17));
#18867=DIRECTION('center_axis',(-1.,0.,0.));
#18868=DIRECTION('ref_axis',(0.,0.,1.));
#18869=DIRECTION('center_axis',(1.,0.,0.));
#18870=DIRECTION('ref_axis',(0.,0.,-1.));
#18871=DIRECTION('center_axis',(-1.,0.,0.));
#18872=DIRECTION('ref_axis',(0.,0.,1.));
#18873=DIRECTION('center_axis',(-1.,0.,0.));
#18874=DIRECTION('ref_axis',(0.,-1.,0.));
#18875=DIRECTION('',(-1.,0.,0.));
#18876=DIRECTION('center_axis',(1.,0.,0.));
#18877=DIRECTION('ref_axis',(0.,-1.,0.));
#18878=DIRECTION('center_axis',(1.,0.,0.));
#18879=DIRECTION('ref_axis',(0.,-1.,0.));
#18880=DIRECTION('center_axis',(-1.,0.,0.));
#18881=DIRECTION('ref_axis',(0.,0.,1.));
#18882=DIRECTION('',(0.707106781186548,0.707106781186547,8.65956056235493E-17));
#18883=DIRECTION('center_axis',(-1.,0.,0.));
#18884=DIRECTION('ref_axis',(0.,-1.,0.));
#18885=DIRECTION('center_axis',(-1.,0.,0.));
#18886=DIRECTION('ref_axis',(0.,-1.,0.));
#18887=DIRECTION('',(-1.,0.,0.));
#18888=DIRECTION('center_axis',(-1.,0.,0.));
#18889=DIRECTION('ref_axis',(0.,0.,1.));
#18890=DIRECTION('center_axis',(-1.,0.,0.));
#18891=DIRECTION('ref_axis',(0.,-1.,0.));
#18892=DIRECTION('',(-0.707106781186551,0.707106781186544,-8.65956056235489E-17));
#18893=DIRECTION('center_axis',(1.,0.,0.));
#18894=DIRECTION('ref_axis',(0.,-1.,0.));
#18895=DIRECTION('center_axis',(-1.,0.,0.));
#18896=DIRECTION('ref_axis',(0.,0.,1.));
#18897=DIRECTION('',(0.707106781186548,0.707106781186547,8.65956056235493E-17));
#18898=DIRECTION('center_axis',(-1.,0.,0.));
#18899=DIRECTION('ref_axis',(0.,-1.,0.));
#18900=DIRECTION('center_axis',(-1.,0.,0.));
#18901=DIRECTION('ref_axis',(0.,-1.,0.));
#18902=DIRECTION('',(-1.,0.,0.));
#18903=DIRECTION('center_axis',(-1.,0.,0.));
#18904=DIRECTION('ref_axis',(0.,0.,1.));
#18905=DIRECTION('center_axis',(-1.,0.,0.));
#18906=DIRECTION('ref_axis',(0.,-1.,0.));
#18907=DIRECTION('',(-0.707106781186551,0.707106781186544,-8.65956056235489E-17));
#18908=DIRECTION('center_axis',(1.,0.,0.));
#18909=DIRECTION('ref_axis',(0.,-1.,0.));
#18910=DIRECTION('center_axis',(-1.,0.,0.));
#18911=DIRECTION('ref_axis',(0.,0.,1.));
#18912=DIRECTION('',(0.707106781186548,0.707106781186547,8.65956056235493E-17));
#18913=DIRECTION('center_axis',(-1.,0.,0.));
#18914=DIRECTION('ref_axis',(0.,-1.,0.));
#18915=DIRECTION('center_axis',(-1.,0.,0.));
#18916=DIRECTION('ref_axis',(0.,-1.,0.));
#18917=DIRECTION('',(-1.,0.,0.));
#18918=DIRECTION('center_axis',(-1.,0.,0.));
#18919=DIRECTION('ref_axis',(0.,0.,1.));
#18920=DIRECTION('center_axis',(-1.,0.,0.));
#18921=DIRECTION('ref_axis',(0.,-1.,0.));
#18922=DIRECTION('',(-0.707106781186551,0.707106781186544,-8.65956056235489E-17));
#18923=DIRECTION('center_axis',(1.,0.,0.));
#18924=DIRECTION('ref_axis',(0.,-1.,0.));
#18925=DIRECTION('center_axis',(-1.,0.,0.));
#18926=DIRECTION('ref_axis',(0.,0.,1.));
#18927=DIRECTION('',(0.707106781186548,0.707106781186547,8.65956056235493E-17));
#18928=DIRECTION('center_axis',(-1.,0.,0.));
#18929=DIRECTION('ref_axis',(0.,-1.,0.));
#18930=DIRECTION('center_axis',(-1.,0.,0.));
#18931=DIRECTION('ref_axis',(0.,-1.,0.));
#18932=DIRECTION('',(-1.,0.,0.));
#18933=DIRECTION('center_axis',(-1.,0.,0.));
#18934=DIRECTION('ref_axis',(0.,0.,1.));
#18935=DIRECTION('center_axis',(-1.,0.,0.));
#18936=DIRECTION('ref_axis',(0.,-1.,0.));
#18937=DIRECTION('',(-0.707106781186551,0.707106781186544,-8.65956056235489E-17));
#18938=DIRECTION('center_axis',(0.,0.,-1.));
#18939=DIRECTION('ref_axis',(0.,-1.,0.));
#18940=DIRECTION('',(0.,-1.,0.));
#18941=DIRECTION('',(-1.,0.,0.));
#18942=DIRECTION('',(-1.,0.,0.));
#18943=DIRECTION('center_axis',(0.,1.,0.));
#18944=DIRECTION('ref_axis',(0.,0.,-1.));
#18945=DIRECTION('',(0.,0.,-1.));
#18946=DIRECTION('',(-1.,0.,0.));
#18947=DIRECTION('center_axis',(0.,0.,1.));
#18948=DIRECTION('ref_axis',(0.,1.,0.));
#18949=DIRECTION('',(0.,1.,0.));
#18950=DIRECTION('',(-1.,0.,0.));
#18951=DIRECTION('center_axis',(0.,-1.,0.));
#18952=DIRECTION('ref_axis',(0.,0.,1.));
#18953=DIRECTION('',(0.,0.,1.));
#18954=DIRECTION('center_axis',(0.,0.,-1.));
#18955=DIRECTION('ref_axis',(0.,-1.,0.));
#18956=DIRECTION('',(0.,-1.,0.));
#18957=DIRECTION('',(-1.,0.,0.));
#18958=DIRECTION('',(-1.,0.,0.));
#18959=DIRECTION('center_axis',(0.,1.,0.));
#18960=DIRECTION('ref_axis',(0.,0.,-1.));
#18961=DIRECTION('',(0.,0.,-1.));
#18962=DIRECTION('',(-1.,0.,0.));
#18963=DIRECTION('center_axis',(0.,0.,1.));
#18964=DIRECTION('ref_axis',(0.,1.,0.));
#18965=DIRECTION('',(0.,1.,0.));
#18966=DIRECTION('',(-1.,0.,0.));
#18967=DIRECTION('center_axis',(0.,-1.,0.));
#18968=DIRECTION('ref_axis',(0.,0.,1.));
#18969=DIRECTION('',(0.,0.,1.));
#18970=DIRECTION('center_axis',(0.,0.,-1.));
#18971=DIRECTION('ref_axis',(0.,-1.,0.));
#18972=DIRECTION('',(0.,-1.,0.));
#18973=DIRECTION('',(-1.,0.,0.));
#18974=DIRECTION('',(-1.,0.,0.));
#18975=DIRECTION('center_axis',(0.,1.,0.));
#18976=DIRECTION('ref_axis',(0.,0.,-1.));
#18977=DIRECTION('',(0.,0.,-1.));
#18978=DIRECTION('',(-1.,0.,0.));
#18979=DIRECTION('center_axis',(0.,0.,1.));
#18980=DIRECTION('ref_axis',(0.,1.,0.));
#18981=DIRECTION('',(0.,1.,0.));
#18982=DIRECTION('',(-1.,0.,0.));
#18983=DIRECTION('center_axis',(0.,-1.,0.));
#18984=DIRECTION('ref_axis',(0.,0.,1.));
#18985=DIRECTION('',(0.,0.,1.));
#18986=DIRECTION('center_axis',(0.,0.,-1.));
#18987=DIRECTION('ref_axis',(0.,-1.,0.));
#18988=DIRECTION('',(0.,-1.,0.));
#18989=DIRECTION('',(-1.,0.,0.));
#18990=DIRECTION('',(-1.,0.,0.));
#18991=DIRECTION('center_axis',(0.,1.,0.));
#18992=DIRECTION('ref_axis',(0.,0.,-1.));
#18993=DIRECTION('',(0.,0.,-1.));
#18994=DIRECTION('',(-1.,0.,0.));
#18995=DIRECTION('center_axis',(0.,0.,1.));
#18996=DIRECTION('ref_axis',(0.,1.,0.));
#18997=DIRECTION('',(0.,1.,0.));
#18998=DIRECTION('',(-1.,0.,0.));
#18999=DIRECTION('center_axis',(0.,-1.,0.));
#19000=DIRECTION('ref_axis',(0.,0.,1.));
#19001=DIRECTION('',(0.,0.,1.));
#19002=DIRECTION('center_axis',(-1.,0.,0.));
#19003=DIRECTION('ref_axis',(0.,0.,-1.));
#19004=DIRECTION('center_axis',(-1.,0.,0.));
#19005=DIRECTION('ref_axis',(0.,0.,-1.));
#19006=DIRECTION('',(-1.,0.,0.));
#19007=DIRECTION('center_axis',(1.,0.,0.));
#19008=DIRECTION('ref_axis',(0.,0.,-1.));
#19009=DIRECTION('center_axis',(1.,0.,0.));
#19010=DIRECTION('ref_axis',(0.,0.,-1.));
#19011=DIRECTION('',(1.,0.,0.));
#19012=DIRECTION('center_axis',(1.,0.,0.));
#19013=DIRECTION('ref_axis',(0.,0.,-1.));
#19014=DIRECTION('center_axis',(1.,0.,0.));
#19015=DIRECTION('ref_axis',(0.,0.,-1.));
#19016=DIRECTION('center_axis',(0.,0.,1.));
#19017=DIRECTION('ref_axis',(0.,1.,0.));
#19018=DIRECTION('',(-1.,0.,0.));
#19019=DIRECTION('',(0.,-1.,0.));
#19020=DIRECTION('center_axis',(0.,-0.707106781186547,0.707106781186548));
#19021=DIRECTION('ref_axis',(0.,0.707106781186548,0.707106781186547));
#19022=DIRECTION('',(-1.,0.,0.));
#19023=DIRECTION('',(0.,-0.707106781186548,-0.707106781186547));
#19024=DIRECTION('center_axis',(0.,-1.,0.));
#19025=DIRECTION('ref_axis',(0.,0.,1.));
#19026=DIRECTION('',(-1.,0.,0.));
#19027=DIRECTION('',(0.,0.,-1.));
#19028=DIRECTION('center_axis',(0.,-0.707106781186548,-0.707106781186548));
#19029=DIRECTION('ref_axis',(0.,-0.707106781186548,0.707106781186548));
#19030=DIRECTION('',(0.,0.707106781186548,-0.707106781186548));
#19031=DIRECTION('center_axis',(1.,0.,0.));
#19032=DIRECTION('ref_axis',(0.,0.,-1.));
#22789=CARTESIAN_POINT('',(0.,0.,0.));
#22790=CARTESIAN_POINT('Origin',(-8.55,6.01214466094067,20.1471446609407));
#22791=CARTESIAN_POINT('',(-8.6,6.9,19.1885786437627));
#22792=CARTESIAN_POINT('',(-8.6,5.68857864376269,20.4));
#22793=CARTESIAN_POINT('',(-8.6,5.97678932188134,20.1117893218813));
#22794=CARTESIAN_POINT('',(-8.5,5.73,20.5));
#22795=CARTESIAN_POINT('',(-8.6,5.68857864376269,20.4));
#22796=CARTESIAN_POINT('',(-8.5,7.,19.23));
#22797=CARTESIAN_POINT('',(-8.5,6.0475,20.1825));
#22798=CARTESIAN_POINT('',(-8.6,6.9,19.1885786437627));
#22799=CARTESIAN_POINT('Origin',(-8.55,-2.865,20.45));
#22800=CARTESIAN_POINT('',(-8.6,-5.68857864376269,20.4));
#22801=CARTESIAN_POINT('',(-8.6,-2.865,20.4));
#22802=CARTESIAN_POINT('',(-8.5,-5.73,20.5));
#22803=CARTESIAN_POINT('',(-8.6,-5.68857864376269,20.4));
#22804=CARTESIAN_POINT('',(-8.5,-2.865,20.5));
#22805=CARTESIAN_POINT('Origin',(-8.55,-6.64714466094067,19.5121446609407));
#22806=CARTESIAN_POINT('',(-8.6,-6.9,19.1885786437627));
#22807=CARTESIAN_POINT('',(-8.6,-6.61178932188135,19.4767893218813));
#22808=CARTESIAN_POINT('',(-8.5,-7.,19.23));
#22809=CARTESIAN_POINT('',(-8.6,-6.9,19.1885786437627));
#22810=CARTESIAN_POINT('',(-8.5,-6.6825,19.5475));
#22811=CARTESIAN_POINT('Origin',(-8.55,-6.95,10.635));
#22812=CARTESIAN_POINT('',(-8.6,-6.9,7.81142135623731));
#22813=CARTESIAN_POINT('',(-8.6,-6.9,10.635));
#22814=CARTESIAN_POINT('',(-8.5,-7.,7.77));
#22815=CARTESIAN_POINT('',(-8.6,-6.9,7.81142135623731));
#22816=CARTESIAN_POINT('',(-8.5,-7.,10.635));
#22817=CARTESIAN_POINT('Origin',(-8.55,-6.01214466094067,6.85285533905933));
#22818=CARTESIAN_POINT('',(-8.6,-5.68857864376269,6.6));
#22819=CARTESIAN_POINT('',(-8.6,-5.97678932188134,6.88821067811866));
#22820=CARTESIAN_POINT('',(-8.5,-5.73,6.5));
#22821=CARTESIAN_POINT('',(-8.6,-5.68857864376269,6.6));
#22822=CARTESIAN_POINT('',(-8.5,-6.0475,6.8175));
#22823=CARTESIAN_POINT('Origin',(-8.55,2.865,6.55));
#22824=CARTESIAN_POINT('',(-8.5,5.73,6.5));
#22825=CARTESIAN_POINT('',(-8.5,2.865,6.5));
#22826=CARTESIAN_POINT('',(-8.6,5.68857864376269,6.6));
#22827=CARTESIAN_POINT('',(-8.6,2.865,6.6));
#22828=CARTESIAN_POINT('',(-8.6,5.68857864376269,6.6));
#22829=CARTESIAN_POINT('Origin',(-8.55,6.64714466094067,7.48785533905933));
#22830=CARTESIAN_POINT('',(-8.5,7.,7.77));
#22831=CARTESIAN_POINT('',(-8.5,6.6825,7.4525));
#22832=CARTESIAN_POINT('',(-8.6,6.9,7.81142135623731));
#22833=CARTESIAN_POINT('',(-8.6,6.61178932188134,7.52321067811866));
#22834=CARTESIAN_POINT('',(-8.6,6.9,7.81142135623731));
#22835=CARTESIAN_POINT('Origin',(-8.55,6.95,16.365));
#22836=CARTESIAN_POINT('',(-8.5,7.,16.365));
#22837=CARTESIAN_POINT('',(-8.6,6.9,16.365));
#22838=CARTESIAN_POINT('Origin',(-7.2,5.73,6.5));
#22839=CARTESIAN_POINT('',(-7.2,5.73,6.5));
#22840=CARTESIAN_POINT('',(-7.2,5.73,6.5));
#22841=CARTESIAN_POINT('',(-7.2,-5.73,6.5));
#22842=CARTESIAN_POINT('',(-7.2,-5.73,6.5));
#22843=CARTESIAN_POINT('',(-7.2,-5.73,6.5));
#22844=CARTESIAN_POINT('Origin',(-7.2,7.,7.77));
#22845=CARTESIAN_POINT('',(-7.2,7.,7.77));
#22846=CARTESIAN_POINT('',(-7.2,7.,7.77));
#22847=CARTESIAN_POINT('',(-7.2,5.73,6.5));
#22848=CARTESIAN_POINT('Origin',(-7.2,7.,19.23));
#22849=CARTESIAN_POINT('',(-7.2,7.,19.23));
#22850=CARTESIAN_POINT('',(-7.2,7.,19.23));
#22851=CARTESIAN_POINT('',(-7.2,7.,7.77));
#22852=CARTESIAN_POINT('Origin',(-7.2,5.73,20.5));
#22853=CARTESIAN_POINT('',(-7.2,5.73,20.5));
#22854=CARTESIAN_POINT('',(-7.2,5.73,20.5));
#22855=CARTESIAN_POINT('',(-7.2,7.,19.23));
#22856=CARTESIAN_POINT('Origin',(-8.6,0.,13.5));
#22857=CARTESIAN_POINT('',(-8.6,-4.116,8.904));
#22858=CARTESIAN_POINT('Origin',(-8.6,-4.596,8.904));
#22859=CARTESIAN_POINT('',(-8.6,5.9,12.));
#22860=CARTESIAN_POINT('',(-8.6,6.6,12.));
#22861=CARTESIAN_POINT('',(-8.6,3.3,12.));
#22862=CARTESIAN_POINT('',(-8.6,6.6,15.));
#22863=CARTESIAN_POINT('',(-8.6,6.6,14.25));
#22864=CARTESIAN_POINT('',(-8.6,5.9,15.));
#22865=CARTESIAN_POINT('',(-8.6,2.95,15.));
#22866=CARTESIAN_POINT('',(-8.6,5.9,12.75));
#22867=CARTESIAN_POINT('',(-8.6,-1.5,6.9));
#22868=CARTESIAN_POINT('',(-8.6,1.5,6.9));
#22869=CARTESIAN_POINT('',(-8.6,0.75,6.9));
#22870=CARTESIAN_POINT('',(-8.6,1.5,7.6));
#22871=CARTESIAN_POINT('',(-8.6,1.5,10.55));
#22872=CARTESIAN_POINT('',(-8.6,-1.5,7.6));
#22873=CARTESIAN_POINT('',(-8.6,-0.75,7.6));
#22874=CARTESIAN_POINT('',(-8.6,-1.5,10.2));
#22875=CARTESIAN_POINT('',(-8.6,-1.5,19.4));
#22876=CARTESIAN_POINT('',(-8.6,1.5,19.4));
#22877=CARTESIAN_POINT('',(-8.6,0.75,19.4));
#22878=CARTESIAN_POINT('',(-8.6,1.5,20.1));
#22879=CARTESIAN_POINT('',(-8.6,1.5,16.8));
#22880=CARTESIAN_POINT('',(-8.6,-1.5,20.1));
#22881=CARTESIAN_POINT('',(-8.6,-0.75,20.1));
#22882=CARTESIAN_POINT('',(-8.6,-1.5,16.45));
#22883=CARTESIAN_POINT('',(-8.6,-6.6,12.));
#22884=CARTESIAN_POINT('',(-8.6,-5.9,12.));
#22885=CARTESIAN_POINT('',(-8.6,-2.95,12.));
#22886=CARTESIAN_POINT('',(-8.6,-5.9,15.));
#22887=CARTESIAN_POINT('',(-8.6,-5.9,14.25));
#22888=CARTESIAN_POINT('',(-8.6,-6.6,15.));
#22889=CARTESIAN_POINT('',(-8.6,-3.3,15.));
#22890=CARTESIAN_POINT('',(-8.6,-6.6,12.75));
#22891=CARTESIAN_POINT('',(-8.6,-6.73678204210959E-16,19.001));
#22892=CARTESIAN_POINT('Origin',(-8.6,0.,13.5));
#22893=CARTESIAN_POINT('',(-8.6,5.076,18.096));
#22894=CARTESIAN_POINT('Origin',(-8.6,4.596,18.096));
#22895=CARTESIAN_POINT('',(-8.6,-4.116,18.096));
#22896=CARTESIAN_POINT('Origin',(-8.6,-4.596,18.096));
#22897=CARTESIAN_POINT('',(-8.6,5.076,8.904));
#22898=CARTESIAN_POINT('Origin',(-8.6,4.596,8.904));
#22899=CARTESIAN_POINT('Origin',(-7.1875,-3.182,10.318));
#22900=CARTESIAN_POINT('',(-7.225,-2.852,10.318));
#22901=CARTESIAN_POINT('Origin',(-7.225,-3.182,10.318));
#22902=CARTESIAN_POINT('',(-7.2,-2.84366666666667,10.318));
#22903=CARTESIAN_POINT('',(-7.1875,-2.8395,10.318));
#22904=CARTESIAN_POINT('Origin',(-7.2,-3.182,10.318));
#22905=CARTESIAN_POINT('Origin',(-7.375,-3.182,10.318));
#22906=CARTESIAN_POINT('',(-7.525,-2.852,10.318));
#22907=CARTESIAN_POINT('',(-7.375,-2.852,10.318));
#22908=CARTESIAN_POINT('Origin',(-7.525,-3.182,10.318));
#22909=CARTESIAN_POINT('Origin',(-7.5375,-3.182,10.318));
#22910=CARTESIAN_POINT('',(-7.55,-2.827,10.318));
#22911=CARTESIAN_POINT('',(-7.5375,-2.8395,10.318));
#22912=CARTESIAN_POINT('Origin',(-7.55,-3.182,10.318));
#22913=CARTESIAN_POINT('Origin',(-7.55,-3.732,10.318));
#22914=CARTESIAN_POINT('',(-7.55,-2.632,10.318));
#22915=CARTESIAN_POINT('Origin',(-7.55,-3.182,10.318));
#22916=CARTESIAN_POINT('Origin',(-7.875,-3.182,10.318));
#22917=CARTESIAN_POINT('',(-8.2,-2.632,10.318));
#22918=CARTESIAN_POINT('',(-7.875,-2.632,10.318));
#22919=CARTESIAN_POINT('Origin',(-8.2,-3.182,10.318));
#22920=CARTESIAN_POINT('Origin',(-7.1875,3.182,10.318));
#22921=CARTESIAN_POINT('',(-7.225,3.512,10.318));
#22922=CARTESIAN_POINT('Origin',(-7.225,3.182,10.318));
#22923=CARTESIAN_POINT('',(-7.2,3.52033333333333,10.318));
#22924=CARTESIAN_POINT('',(-7.1875,3.5245,10.318));
#22925=CARTESIAN_POINT('Origin',(-7.2,3.182,10.318));
#22926=CARTESIAN_POINT('Origin',(-7.375,3.182,10.318));
#22927=CARTESIAN_POINT('',(-7.525,3.512,10.318));
#22928=CARTESIAN_POINT('',(-7.375,3.512,10.318));
#22929=CARTESIAN_POINT('Origin',(-7.525,3.182,10.318));
#22930=CARTESIAN_POINT('Origin',(-7.5375,3.182,10.318));
#22931=CARTESIAN_POINT('',(-7.55,3.537,10.318));
#22932=CARTESIAN_POINT('',(-7.5375,3.5245,10.318));
#22933=CARTESIAN_POINT('Origin',(-7.55,3.182,10.318));
#22934=CARTESIAN_POINT('Origin',(-7.55,2.632,10.318));
#22935=CARTESIAN_POINT('',(-7.55,3.732,10.318));
#22936=CARTESIAN_POINT('Origin',(-7.55,3.182,10.318));
#22937=CARTESIAN_POINT('Origin',(-7.875,3.182,10.318));
#22938=CARTESIAN_POINT('',(-8.2,3.732,10.318));
#22939=CARTESIAN_POINT('',(-7.875,3.732,10.318));
#22940=CARTESIAN_POINT('Origin',(-8.2,3.182,10.318));
#22941=CARTESIAN_POINT('Origin',(-7.1875,-3.182,16.682));
#22942=CARTESIAN_POINT('',(-7.225,-2.852,16.682));
#22943=CARTESIAN_POINT('Origin',(-7.225,-3.182,16.682));
#22944=CARTESIAN_POINT('',(-7.2,-2.84366666666667,16.682));
#22945=CARTESIAN_POINT('',(-7.1875,-2.8395,16.682));
#22946=CARTESIAN_POINT('Origin',(-7.2,-3.182,16.682));
#22947=CARTESIAN_POINT('Origin',(-7.375,-3.182,16.682));
#22948=CARTESIAN_POINT('',(-7.525,-2.852,16.682));
#22949=CARTESIAN_POINT('',(-7.375,-2.852,16.682));
#22950=CARTESIAN_POINT('Origin',(-7.525,-3.182,16.682));
#22951=CARTESIAN_POINT('Origin',(-7.5375,-3.182,16.682));
#22952=CARTESIAN_POINT('',(-7.55,-2.827,16.682));
#22953=CARTESIAN_POINT('',(-7.5375,-2.8395,16.682));
#22954=CARTESIAN_POINT('Origin',(-7.55,-3.182,16.682));
#22955=CARTESIAN_POINT('Origin',(-7.55,-3.732,16.682));
#22956=CARTESIAN_POINT('',(-7.55,-2.632,16.682));
#22957=CARTESIAN_POINT('Origin',(-7.55,-3.182,16.682));
#22958=CARTESIAN_POINT('Origin',(-7.875,-3.182,16.682));
#22959=CARTESIAN_POINT('',(-8.2,-2.632,16.682));
#22960=CARTESIAN_POINT('',(-7.875,-2.632,16.682));
#22961=CARTESIAN_POINT('Origin',(-8.2,-3.182,16.682));
#22962=CARTESIAN_POINT('Origin',(-7.1875,3.182,16.682));
#22963=CARTESIAN_POINT('',(-7.225,3.512,16.682));
#22964=CARTESIAN_POINT('Origin',(-7.225,3.182,16.682));
#22965=CARTESIAN_POINT('',(-7.2,3.52033333333333,16.682));
#22966=CARTESIAN_POINT('',(-7.1875,3.5245,16.682));
#22967=CARTESIAN_POINT('Origin',(-7.2,3.182,16.682));
#22968=CARTESIAN_POINT('Origin',(-7.375,3.182,16.682));
#22969=CARTESIAN_POINT('',(-7.525,3.512,16.682));
#22970=CARTESIAN_POINT('',(-7.375,3.512,16.682));
#22971=CARTESIAN_POINT('Origin',(-7.525,3.182,16.682));
#22972=CARTESIAN_POINT('Origin',(-7.5375,3.182,16.682));
#22973=CARTESIAN_POINT('',(-7.55,3.537,16.682));
#22974=CARTESIAN_POINT('',(-7.5375,3.5245,16.682));
#22975=CARTESIAN_POINT('Origin',(-7.55,3.182,16.682));
#22976=CARTESIAN_POINT('Origin',(-7.55,2.632,16.682));
#22977=CARTESIAN_POINT('',(-7.55,3.732,16.682));
#22978=CARTESIAN_POINT('Origin',(-7.55,3.182,16.682));
#22979=CARTESIAN_POINT('Origin',(-7.875,3.182,16.682));
#22980=CARTESIAN_POINT('',(-8.2,3.732,16.682));
#22981=CARTESIAN_POINT('',(-7.875,3.732,16.682));
#22982=CARTESIAN_POINT('Origin',(-8.2,3.182,16.682));
#22983=CARTESIAN_POINT('Origin',(-7.19,-4.596,8.904));
#22984=CARTESIAN_POINT('',(-7.23,-4.146,8.904));
#22985=CARTESIAN_POINT('Origin',(-7.23,-4.596,8.904));
#22986=CARTESIAN_POINT('',(-7.2,-4.116,8.904));
#22987=CARTESIAN_POINT('',(-7.19,-4.106,8.904));
#22988=CARTESIAN_POINT('Origin',(-7.2,-4.596,8.904));
#22989=CARTESIAN_POINT('Origin',(-7.9,-4.596,8.904));
#22990=CARTESIAN_POINT('',(-8.57,-4.146,8.904));
#22991=CARTESIAN_POINT('',(-7.9,-4.146,8.904));
#22992=CARTESIAN_POINT('Origin',(-8.57,-4.596,8.904));
#22993=CARTESIAN_POINT('Origin',(-8.61,-4.596,8.904));
#22994=CARTESIAN_POINT('',(-8.61,-4.106,8.904));
#22995=CARTESIAN_POINT('Origin',(-7.19,4.596,8.904));
#22996=CARTESIAN_POINT('',(-7.23,5.046,8.904));
#22997=CARTESIAN_POINT('Origin',(-7.23,4.596,8.904));
#22998=CARTESIAN_POINT('',(-7.2,5.076,8.904));
#22999=CARTESIAN_POINT('',(-7.19,5.086,8.904));
#23000=CARTESIAN_POINT('Origin',(-7.2,4.596,8.904));
#23001=CARTESIAN_POINT('Origin',(-7.9,4.596,8.904));
#23002=CARTESIAN_POINT('',(-8.57,5.046,8.904));
#23003=CARTESIAN_POINT('',(-7.9,5.046,8.904));
#23004=CARTESIAN_POINT('Origin',(-8.57,4.596,8.904));
#23005=CARTESIAN_POINT('Origin',(-8.61,4.596,8.904));
#23006=CARTESIAN_POINT('',(-8.61,5.086,8.904));
#23007=CARTESIAN_POINT('Origin',(-7.19,-4.596,18.096));
#23008=CARTESIAN_POINT('',(-7.23,-4.146,18.096));
#23009=CARTESIAN_POINT('Origin',(-7.23,-4.596,18.096));
#23010=CARTESIAN_POINT('',(-7.2,-4.116,18.096));
#23011=CARTESIAN_POINT('',(-7.19,-4.106,18.096));
#23012=CARTESIAN_POINT('Origin',(-7.2,-4.596,18.096));
#23013=CARTESIAN_POINT('Origin',(-7.9,-4.596,18.096));
#23014=CARTESIAN_POINT('',(-8.57,-4.146,18.096));
#23015=CARTESIAN_POINT('',(-7.9,-4.146,18.096));
#23016=CARTESIAN_POINT('Origin',(-8.57,-4.596,18.096));
#23017=CARTESIAN_POINT('Origin',(-8.61,-4.596,18.096));
#23018=CARTESIAN_POINT('',(-8.61,-4.106,18.096));
#23019=CARTESIAN_POINT('Origin',(-7.19,4.596,18.096));
#23020=CARTESIAN_POINT('',(-7.23,5.046,18.096));
#23021=CARTESIAN_POINT('Origin',(-7.23,4.596,18.096));
#23022=CARTESIAN_POINT('',(-7.2,5.076,18.096));
#23023=CARTESIAN_POINT('',(-7.19,5.086,18.096));
#23024=CARTESIAN_POINT('Origin',(-7.2,4.596,18.096));
#23025=CARTESIAN_POINT('Origin',(-7.9,4.596,18.096));
#23026=CARTESIAN_POINT('',(-8.57,5.046,18.096));
#23027=CARTESIAN_POINT('',(-7.9,5.046,18.096));
#23028=CARTESIAN_POINT('Origin',(-8.57,4.596,18.096));
#23029=CARTESIAN_POINT('Origin',(-8.61,4.596,18.096));
#23030=CARTESIAN_POINT('',(-8.61,5.086,18.096));
#23031=CARTESIAN_POINT('Origin',(-7.2,6.6,12.));
#23032=CARTESIAN_POINT('',(-7.2,6.6,12.));
#23033=CARTESIAN_POINT('',(-7.2,5.9,12.));
#23034=CARTESIAN_POINT('',(-7.2,3.3,12.));
#23035=CARTESIAN_POINT('',(-7.2,6.6,12.));
#23036=CARTESIAN_POINT('',(-7.2,5.9,12.));
#23037=CARTESIAN_POINT('Origin',(-7.2,6.6,15.));
#23038=CARTESIAN_POINT('',(-7.2,6.6,15.));
#23039=CARTESIAN_POINT('',(-7.2,6.6,14.25));
#23040=CARTESIAN_POINT('',(-7.2,6.6,15.));
#23041=CARTESIAN_POINT('Origin',(-7.2,5.9,15.));
#23042=CARTESIAN_POINT('',(-7.2,5.9,15.));
#23043=CARTESIAN_POINT('',(-7.2,2.95,15.));
#23044=CARTESIAN_POINT('',(-7.2,5.9,15.));
#23045=CARTESIAN_POINT('Origin',(-7.2,5.9,12.));
#23046=CARTESIAN_POINT('',(-7.2,5.9,12.75));
#23047=CARTESIAN_POINT('Origin',(-7.2,1.5,6.9));
#23048=CARTESIAN_POINT('',(-7.2,1.5,6.9));
#23049=CARTESIAN_POINT('',(-7.2,-1.5,6.9));
#23050=CARTESIAN_POINT('',(-7.2,0.75,6.9));
#23051=CARTESIAN_POINT('',(-7.2,1.5,6.9));
#23052=CARTESIAN_POINT('',(-7.2,-1.5,6.9));
#23053=CARTESIAN_POINT('Origin',(-7.2,1.5,7.6));
#23054=CARTESIAN_POINT('',(-7.2,1.5,7.6));
#23055=CARTESIAN_POINT('',(-7.2,1.5,10.55));
#23056=CARTESIAN_POINT('',(-7.2,1.5,7.6));
#23057=CARTESIAN_POINT('Origin',(-7.2,-1.5,7.6));
#23058=CARTESIAN_POINT('',(-7.2,-1.5,7.6));
#23059=CARTESIAN_POINT('',(-7.2,-0.75,7.6));
#23060=CARTESIAN_POINT('',(-7.2,-1.5,7.6));
#23061=CARTESIAN_POINT('Origin',(-7.2,-1.5,6.9));
#23062=CARTESIAN_POINT('',(-7.2,-1.5,10.2));
#23063=CARTESIAN_POINT('Origin',(-7.2,1.5,19.4));
#23064=CARTESIAN_POINT('',(-7.2,1.5,19.4));
#23065=CARTESIAN_POINT('',(-7.2,-1.5,19.4));
#23066=CARTESIAN_POINT('',(-7.2,0.75,19.4));
#23067=CARTESIAN_POINT('',(-7.2,1.5,19.4));
#23068=CARTESIAN_POINT('',(-7.2,-1.5,19.4));
#23069=CARTESIAN_POINT('Origin',(-7.2,1.5,20.1));
#23070=CARTESIAN_POINT('',(-7.2,1.5,20.1));
#23071=CARTESIAN_POINT('',(-7.2,1.5,16.8));
#23072=CARTESIAN_POINT('',(-7.2,1.5,20.1));
#23073=CARTESIAN_POINT('Origin',(-7.2,-1.5,20.1));
#23074=CARTESIAN_POINT('',(-7.2,-1.5,20.1));
#23075=CARTESIAN_POINT('',(-7.2,-0.75,20.1));
#23076=CARTESIAN_POINT('',(-7.2,-1.5,20.1));
#23077=CARTESIAN_POINT('Origin',(-7.2,-1.5,19.4));
#23078=CARTESIAN_POINT('',(-7.2,-1.5,16.45));
#23079=CARTESIAN_POINT('Origin',(-7.2,-5.9,12.));
#23080=CARTESIAN_POINT('',(-7.2,-5.9,12.));
#23081=CARTESIAN_POINT('',(-7.2,-6.6,12.));
#23082=CARTESIAN_POINT('',(-7.2,-2.95,12.));
#23083=CARTESIAN_POINT('',(-7.2,-5.9,12.));
#23084=CARTESIAN_POINT('',(-7.2,-6.6,12.));
#23085=CARTESIAN_POINT('Origin',(-7.2,-5.9,15.));
#23086=CARTESIAN_POINT('',(-7.2,-5.9,15.));
#23087=CARTESIAN_POINT('',(-7.2,-5.9,14.25));
#23088=CARTESIAN_POINT('',(-7.2,-5.9,15.));
#23089=CARTESIAN_POINT('Origin',(-7.2,-6.6,15.));
#23090=CARTESIAN_POINT('',(-7.2,-6.6,15.));
#23091=CARTESIAN_POINT('',(-7.2,-3.3,15.));
#23092=CARTESIAN_POINT('',(-7.2,-6.6,15.));
#23093=CARTESIAN_POINT('Origin',(-7.2,-6.6,12.));
#23094=CARTESIAN_POINT('',(-7.2,-6.6,12.75));
#23095=CARTESIAN_POINT('Origin',(-7.2,0.,13.5));
#23096=CARTESIAN_POINT('',(-7.2,-2.44929359829471E-16,15.5));
#23097=CARTESIAN_POINT('Origin',(-7.2,0.,13.5));
#23098=CARTESIAN_POINT('',(-8.2,-2.44929359829471E-16,15.5));
#23099=CARTESIAN_POINT('',(-7.2,2.44929359829471E-16,15.5));
#23100=CARTESIAN_POINT('Origin',(-8.2,0.,13.5));
#23101=CARTESIAN_POINT('Origin',(-8.6,0.,13.5));
#23102=CARTESIAN_POINT('',(-8.2,-6.73678204210959E-16,19.001));
#23103=CARTESIAN_POINT('',(-8.6,-6.73678204210959E-16,19.001));
#23104=CARTESIAN_POINT('Origin',(-8.2,0.,13.5));
#23105=CARTESIAN_POINT('Origin',(-8.2,0.,13.5));
#23106=CARTESIAN_POINT('Origin',(-7.2,-5.73,20.5));
#23107=CARTESIAN_POINT('',(-7.2,-5.73,20.5));
#23108=CARTESIAN_POINT('',(-7.2,-5.73,20.5));
#23109=CARTESIAN_POINT('',(-7.2,5.73,20.5));
#23110=CARTESIAN_POINT('Origin',(-7.2,-7.,19.23));
#23111=CARTESIAN_POINT('',(-7.2,-7.,19.23));
#23112=CARTESIAN_POINT('',(-7.2,-7.,19.23));
#23113=CARTESIAN_POINT('',(-7.2,-5.73,20.5));
#23114=CARTESIAN_POINT('Origin',(-7.2,-7.,7.77));
#23115=CARTESIAN_POINT('',(-7.2,-7.,7.77));
#23116=CARTESIAN_POINT('',(-7.2,-7.,7.77));
#23117=CARTESIAN_POINT('',(-7.2,-7.,19.23));
#23118=CARTESIAN_POINT('Origin',(-7.2,-5.73,6.5));
#23119=CARTESIAN_POINT('',(-7.2,-7.,7.77));
#23120=CARTESIAN_POINT('Origin',(-7.2,0.,13.5));
#86393=UNCERTAINTY_MEASURE_WITH_UNIT(LENGTH_MEASURE(0.001),#86430,
'DISTANCE_ACCURACY_VALUE',
'Maximum model space distance between geometric entities at asserted c
onnectivities');
#86409=UNCERTAINTY_MEASURE_WITH_UNIT(LENGTH_MEASURE(0.001),#86430,
'DISTANCE_ACCURACY_VALUE',
'Maximum model space distance between geometric entities at asserted c
onnectivities');
#86413=(
GEOMETRIC_REPRESENTATION_CONTEXT(3)
GLOBAL_UNCERTAINTY_ASSIGNED_CONTEXT((#86393))
GLOBAL_UNIT_ASSIGNED_CONTEXT((#86430,#86432,#86433))
REPRESENTATION_CONTEXT('','3D')
);
#86429=(
GEOMETRIC_REPRESENTATION_CONTEXT(3)
GLOBAL_UNCERTAINTY_ASSIGNED_CONTEXT((#86409))
GLOBAL_UNIT_ASSIGNED_CONTEXT((#86430,#86432,#86433))
REPRESENTATION_CONTEXT('','3D')
);
#86430=(
LENGTH_UNIT()
NAMED_UNIT(*)
SI_UNIT(.CENTI.,.METRE.)
);
#86432=(
NAMED_UNIT(*)
PLANE_ANGLE_UNIT()
SI_UNIT($,.RADIAN.)
);
#86433=(
NAMED_UNIT(*)
SI_UNIT($,.STERADIAN.)
SOLID_ANGLE_UNIT()
);
#86437=SHAPE_DEFINITION_REPRESENTATION(#86456,#86504);
#86456=PRODUCT_DEFINITION_SHAPE('',$,#86524);
#86504=SHAPE_REPRESENTATION('',(#16305),#86413);
#86520=PRODUCT_DEFINITION_CONTEXT('part definition',#86579,'design');
#86524=PRODUCT_DEFINITION('IEC71 B5 Input Motor Flange',
'IEC71 B5 Input Motor Flange',#86543,#86520);
#86543=PRODUCT_DEFINITION_FORMATION('',$,#86584);
#86579=APPLICATION_CONTEXT(
'Core Data for Automotive Mechanical Design Process');
#86580=PRODUCT_CONTEXT('part definition',#86579,'mechanical');
#86584=PRODUCT('IEC71 B5 Input Motor Flange',
'IEC71 B5 Input Motor Flange',$,(#86580));
#86603=PRESENTATION_STYLE_ASSIGNMENT((#86621));
#86621=SURFACE_STYLE_USAGE(.BOTH.,#86639);
#86639=SURFACE_SIDE_STYLE('',(#86657));
#86657=SURFACE_STYLE_FILL_AREA(#86675);
#86675=FILL_AREA_STYLE('Opaque(198,201,205)',(#86693));
#86693=FILL_AREA_STYLE_COLOUR('Opaque(198,201,205)',#86711);
#86711=COLOUR_RGB('Opaque(198,201,205)', 0.31764706, 0.68627451, 0.89019608);
ENDSEC;
END-ISO-10303-21;
